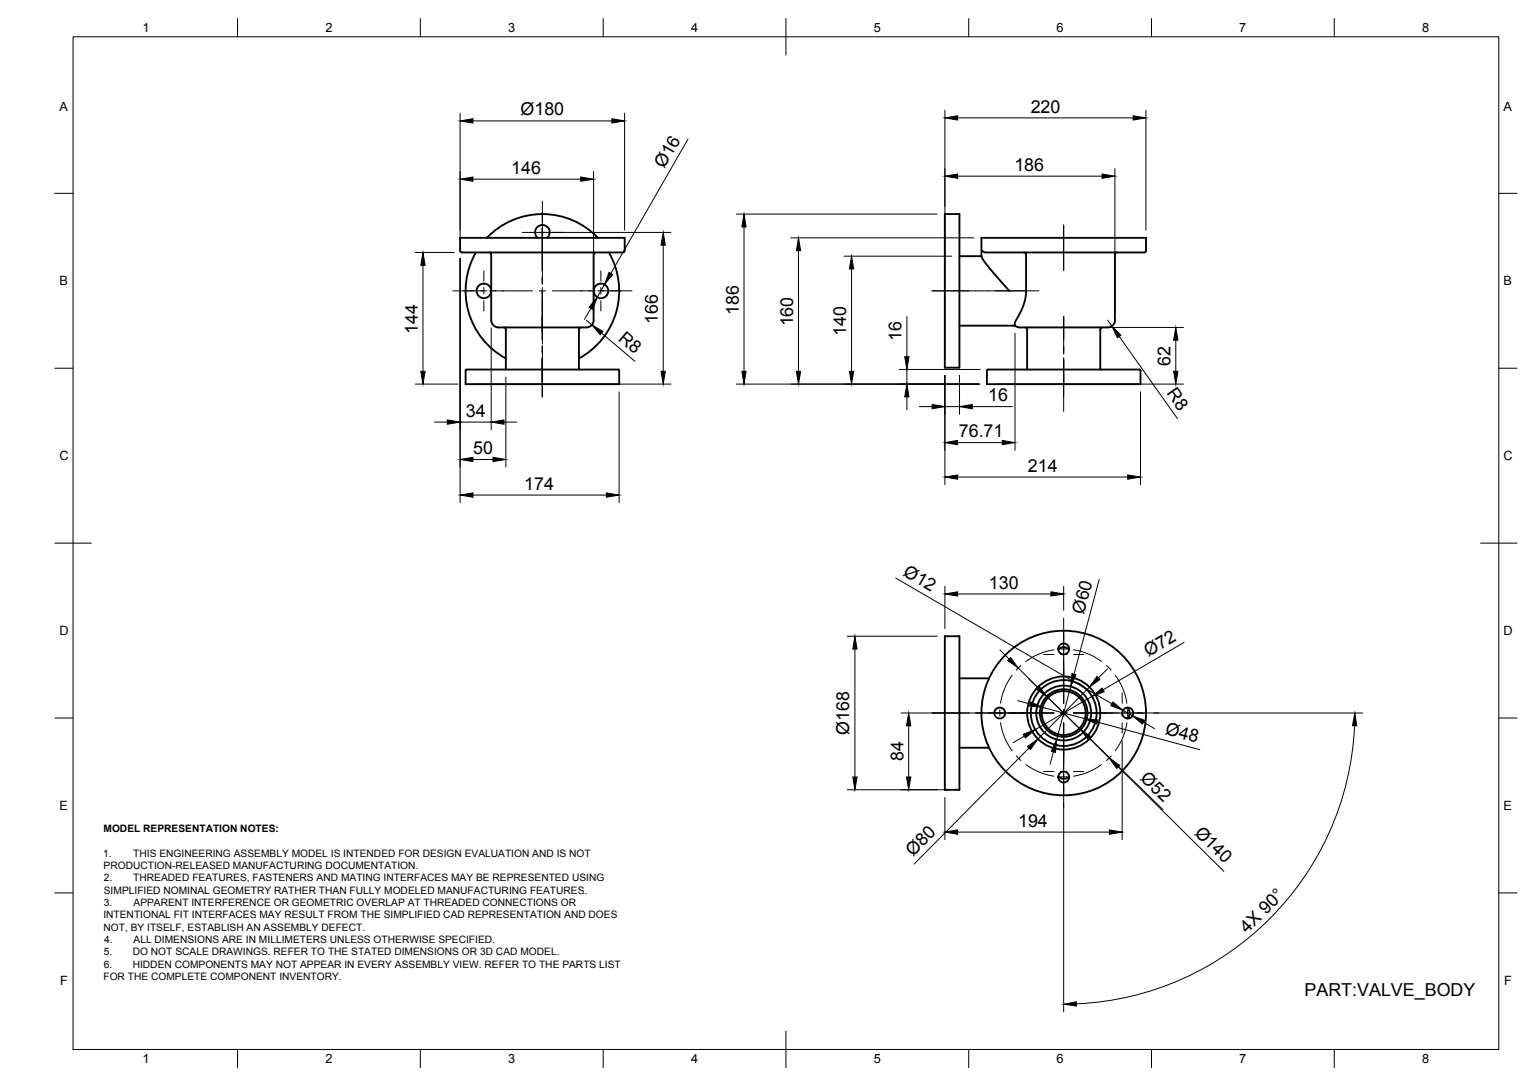
ISO-10303-21;
HEADER;
/* Generated by software containing ST-Developer
 * from STEP Tools, Inc. (www.steptools.com) 
 */

FILE_DESCRIPTION(
/* description */ (''),
/* implementation_level */ '2;1');

FILE_NAME(
/* name */ 'VALVE_BODY.step',
/* time_stamp */ '2026-10-04T02:10:06-07:00',
/* author */ (''),
/* organization */ (''),
/* preprocessor_version */ 'ST-DEVELOPER v20.2',
/* originating_system */ 'Autodesk Translation Framework v15.15.0.0',
/* authorisation */ '');

FILE_SCHEMA (('AUTOMOTIVE_DESIGN { 1 0 10303 214 3 1 1 }'));
ENDSEC;

DATA;
#10=MECHANICAL_DESIGN_GEOMETRIC_PRESENTATION_REPRESENTATION('',(#141),#9668);
#119=SHAPE_REPRESENTATION_RELATIONSHIP('SRR','None',#9712,#130);
#130=ADVANCED_BREP_SHAPE_REPRESENTATION('',(#152),#9657);
#141=STYLED_ITEM('',(#9775),#152);
#152=MANIFOLD_SOLID_BREP('Body1',#3881);
#163=CONICAL_SURFACE('',#4037,30.,0.785398163397447);
#164=CONICAL_SURFACE('',#4125,1000.,1.02974425867666);
#195=FACE_BOUND('',#1037,.T.);
#196=FACE_BOUND('',#1038,.T.);
#197=FACE_BOUND('',#1039,.T.);
#198=FACE_BOUND('',#1041,.T.);
#199=FACE_BOUND('',#1045,.T.);
#200=FACE_BOUND('',#1048,.T.);
#201=FACE_BOUND('',#1049,.T.);
#202=FACE_BOUND('',#1050,.T.);
#203=FACE_BOUND('',#1051,.T.);
#204=FACE_BOUND('',#1052,.T.);
#205=FACE_BOUND('',#1055,.T.);
#206=FACE_BOUND('',#1056,.T.);
#207=FACE_BOUND('',#1057,.T.);
#208=FACE_BOUND('',#1058,.T.);
#209=FACE_BOUND('',#1059,.T.);
#210=FACE_BOUND('',#1063,.T.);
#211=FACE_BOUND('',#1068,.T.);
#212=FACE_BOUND('',#1069,.T.);
#213=FACE_BOUND('',#1070,.T.);
#214=FACE_BOUND('',#1071,.T.);
#215=FACE_BOUND('',#1072,.T.);
#216=FACE_BOUND('',#1075,.T.);
#217=FACE_BOUND('',#1077,.T.);
#218=FACE_BOUND('',#1079,.T.);
#219=FACE_BOUND('',#1083,.T.);
#220=FACE_BOUND('',#1084,.T.);
#221=FACE_BOUND('',#1085,.T.);
#222=FACE_BOUND('',#1086,.T.);
#223=FACE_BOUND('',#1087,.T.);
#224=FACE_BOUND('',#1089,.T.);
#225=FACE_BOUND('',#1090,.T.);
#226=FACE_BOUND('',#1091,.T.);
#227=FACE_BOUND('',#1092,.T.);
#228=FACE_BOUND('',#1093,.T.);
#268=PLANE('',#4028);
#269=PLANE('',#4034);
#270=PLANE('',#4042);
#271=PLANE('',#4046);
#272=PLANE('',#4055);
#273=PLANE('',#4068);
#274=PLANE('',#4078);
#275=PLANE('',#4088);
#276=PLANE('',#4092);
#277=PLANE('',#4099);
#278=PLANE('',#4104);
#279=PLANE('',#4111);
#280=PLANE('',#4112);
#371=LINE('',#5637,#562);
#372=LINE('',#5688,#563);
#373=LINE('',#5690,#564);
#374=LINE('',#5995,#565);
#375=LINE('',#5997,#566);
#376=LINE('',#6015,#567);
#377=LINE('',#6018,#568);
#378=LINE('',#6025,#569);
#379=LINE('',#6040,#570);
#380=LINE('',#6059,#571);
#381=LINE('',#6078,#572);
#382=LINE('',#6080,#573);
#383=LINE('',#6082,#574);
#384=LINE('',#6084,#575);
#385=LINE('',#6102,#576);
#386=LINE('',#6109,#577);
#387=LINE('',#6190,#578);
#388=LINE('',#6213,#579);
#389=LINE('',#6214,#580);
#390=LINE('',#6216,#581);
#391=LINE('',#6218,#582);
#392=LINE('',#6220,#583);
#393=LINE('',#6222,#584);
#394=LINE('',#6224,#585);
#395=LINE('',#6226,#586);
#396=LINE('',#6228,#587);
#397=LINE('',#6230,#588);
#398=LINE('',#6232,#589);
#399=LINE('',#6234,#590);
#400=LINE('',#6236,#591);
#401=LINE('',#6239,#592);
#402=LINE('',#6245,#593);
#403=LINE('',#6247,#594);
#404=LINE('',#6249,#595);
#405=LINE('',#6251,#596);
#562=VECTOR('',#4483,18.3303029094034);
#563=VECTOR('',#4484,38.);
#564=VECTOR('',#4487,18.3303193041542);
#565=VECTOR('',#4504,15.6464703888607);
#566=VECTOR('',#4505,15.6464703888607);
#567=VECTOR('',#4526,30.);
#568=VECTOR('',#4529,26.);
#569=VECTOR('',#4538,23.9999999999998);
#570=VECTOR('',#4555,83.9999999999998);
#571=VECTOR('',#4576,39.9999999999999);
#572=VECTOR('',#4603,56.0000000000001);
#573=VECTOR('',#4606,7.94448724536034);
#574=VECTOR('',#4607,90.0000000000003);
#575=VECTOR('',#4610,7.94448724536034);
#576=VECTOR('',#4629,39.999999999998);
#577=VECTOR('',#4638,44.0000000000001);
#578=VECTOR('',#4653,84.);
#579=VECTOR('',#4680,40.0090835271346);
#580=VECTOR('',#4681,40.011431530049);
#581=VECTOR('',#4684,42.);
#582=VECTOR('',#4687,42.);
#583=VECTOR('',#4690,24.);
#584=VECTOR('',#4693,8.);
#585=VECTOR('',#4696,8.);
#586=VECTOR('',#4699,8.);
#587=VECTOR('',#4702,8.);
#588=VECTOR('',#4705,8.);
#589=VECTOR('',#4708,8.);
#590=VECTOR('',#4711,8.);
#591=VECTOR('',#4714,8.);
#592=VECTOR('',#4717,6.00000000000001);
#593=VECTOR('',#4724,1000.);
#594=VECTOR('',#4727,6.00000000000001);
#595=VECTOR('',#4730,6.00000000000001);
#596=VECTOR('',#4733,6.00000000000001);
#753=CYLINDRICAL_SURFACE('',#4020,38.);
#754=CYLINDRICAL_SURFACE('',#4040,26.);
#755=CYLINDRICAL_SURFACE('',#4044,23.9999999999998);
#756=CYLINDRICAL_SURFACE('',#4052,83.9999999999998);
#757=CYLINDRICAL_SURFACE('',#4062,39.9999999999999);
#758=CYLINDRICAL_SURFACE('',#4075,56.0000000000001);
#759=CYLINDRICAL_SURFACE('',#4076,90.0000000000003);
#760=CYLINDRICAL_SURFACE('',#4084,39.999999999998);
#761=CYLINDRICAL_SURFACE('',#4090,44.0000000000001);
#762=CYLINDRICAL_SURFACE('',#4096,84.);
#763=CYLINDRICAL_SURFACE('',#4110,56.);
#764=CYLINDRICAL_SURFACE('',#4113,24.);
#765=CYLINDRICAL_SURFACE('',#4114,8.);
#766=CYLINDRICAL_SURFACE('',#4115,8.);
#767=CYLINDRICAL_SURFACE('',#4116,8.);
#768=CYLINDRICAL_SURFACE('',#4117,8.);
#769=CYLINDRICAL_SURFACE('',#4118,8.);
#770=CYLINDRICAL_SURFACE('',#4119,8.);
#771=CYLINDRICAL_SURFACE('',#4120,8.);
#772=CYLINDRICAL_SURFACE('',#4121,8.);
#773=CYLINDRICAL_SURFACE('',#4122,6.00000000000001);
#774=CYLINDRICAL_SURFACE('',#4126,6.00000000000001);
#775=CYLINDRICAL_SURFACE('',#4127,6.00000000000001);
#776=CYLINDRICAL_SURFACE('',#4128,6.00000000000001);
#777=CYLINDRICAL_SURFACE('',#4129,30.);
#778=CYLINDRICAL_SURFACE('',#4130,30.);
#810=FACE_OUTER_BOUND('',#1033,.T.);
#811=FACE_OUTER_BOUND('',#1034,.T.);
#812=FACE_OUTER_BOUND('',#1035,.T.);
#813=FACE_OUTER_BOUND('',#1036,.T.);
#814=FACE_OUTER_BOUND('',#1040,.T.);
#815=FACE_OUTER_BOUND('',#1042,.T.);
#816=FACE_OUTER_BOUND('',#1043,.T.);
#817=FACE_OUTER_BOUND('',#1044,.T.);
#818=FACE_OUTER_BOUND('',#1046,.T.);
#819=FACE_OUTER_BOUND('',#1047,.T.);
#820=FACE_OUTER_BOUND('',#1053,.T.);
#821=FACE_OUTER_BOUND('',#1054,.T.);
#822=FACE_OUTER_BOUND('',#1060,.T.);
#823=FACE_OUTER_BOUND('',#1061,.T.);
#824=FACE_OUTER_BOUND('',#1062,.T.);
#825=FACE_OUTER_BOUND('',#1064,.T.);
#826=FACE_OUTER_BOUND('',#1065,.T.);
#827=FACE_OUTER_BOUND('',#1066,.T.);
#828=FACE_OUTER_BOUND('',#1067,.T.);
#829=FACE_OUTER_BOUND('',#1073,.T.);
#830=FACE_OUTER_BOUND('',#1074,.T.);
#831=FACE_OUTER_BOUND('',#1076,.T.);
#832=FACE_OUTER_BOUND('',#1078,.T.);
#833=FACE_OUTER_BOUND('',#1080,.T.);
#834=FACE_OUTER_BOUND('',#1081,.T.);
#835=FACE_OUTER_BOUND('',#1082,.T.);
#836=FACE_OUTER_BOUND('',#1088,.T.);
#837=FACE_OUTER_BOUND('',#1094,.T.);
#838=FACE_OUTER_BOUND('',#1095,.T.);
#839=FACE_OUTER_BOUND('',#1096,.T.);
#840=FACE_OUTER_BOUND('',#1097,.T.);
#841=FACE_OUTER_BOUND('',#1098,.T.);
#842=FACE_OUTER_BOUND('',#1099,.T.);
#843=FACE_OUTER_BOUND('',#1100,.T.);
#844=FACE_OUTER_BOUND('',#1101,.T.);
#845=FACE_OUTER_BOUND('',#1102,.T.);
#846=FACE_OUTER_BOUND('',#1103,.T.);
#847=FACE_OUTER_BOUND('',#1104,.T.);
#848=FACE_OUTER_BOUND('',#1105,.T.);
#849=FACE_OUTER_BOUND('',#1106,.T.);
#850=FACE_OUTER_BOUND('',#1107,.T.);
#851=FACE_OUTER_BOUND('',#1108,.T.);
#852=FACE_OUTER_BOUND('',#1109,.T.);
#853=FACE_OUTER_BOUND('',#1110,.T.);
#854=FACE_OUTER_BOUND('',#1111,.T.);
#855=FACE_OUTER_BOUND('',#1112,.T.);
#856=FACE_OUTER_BOUND('',#1113,.T.);
#857=FACE_OUTER_BOUND('',#1114,.T.);
#1033=EDGE_LOOP('',(#2541,#2542,#2543,#2544,#2545));
#1034=EDGE_LOOP('',(#2546,#2547,#2548,#2549,#2550,#2551,#2552,#2553,#2554,
#2555,#2556,#2557));
#1035=EDGE_LOOP('',(#2558,#2559,#2560,#2561,#2562,#2563,#2564,#2565,#2566));
#1036=EDGE_LOOP('',(#2567,#2568,#2569,#2570,#2571,#2572,#2573));
#1037=EDGE_LOOP('',(#2574));
#1038=EDGE_LOOP('',(#2575));
#1039=EDGE_LOOP('',(#2576));
#1040=EDGE_LOOP('',(#2577));
#1041=EDGE_LOOP('',(#2578));
#1042=EDGE_LOOP('',(#2579,#2580,#2581,#2582,#2583));
#1043=EDGE_LOOP('',(#2584,#2585,#2586,#2587,#2588));
#1044=EDGE_LOOP('',(#2589));
#1045=EDGE_LOOP('',(#2590));
#1046=EDGE_LOOP('',(#2591,#2592,#2593,#2594));
#1047=EDGE_LOOP('',(#2595));
#1048=EDGE_LOOP('',(#2596));
#1049=EDGE_LOOP('',(#2597));
#1050=EDGE_LOOP('',(#2598));
#1051=EDGE_LOOP('',(#2599));
#1052=EDGE_LOOP('',(#2600));
#1053=EDGE_LOOP('',(#2601,#2602,#2603,#2604,#2605));
#1054=EDGE_LOOP('',(#2606));
#1055=EDGE_LOOP('',(#2607));
#1056=EDGE_LOOP('',(#2608));
#1057=EDGE_LOOP('',(#2609));
#1058=EDGE_LOOP('',(#2610));
#1059=EDGE_LOOP('',(#2611));
#1060=EDGE_LOOP('',(#2612,#2613,#2614,#2615,#2616));
#1061=EDGE_LOOP('',(#2617,#2618,#2619,#2620,#2621));
#1062=EDGE_LOOP('',(#2622));
#1063=EDGE_LOOP('',(#2623));
#1064=EDGE_LOOP('',(#2624,#2625,#2626,#2627,#2628,#2629,#2630));
#1065=EDGE_LOOP('',(#2631,#2632,#2633,#2634,#2635,#2636,#2637,#2638,#2639));
#1066=EDGE_LOOP('',(#2640,#2641,#2642,#2643,#2644,#2645,#2646,#2647));
#1067=EDGE_LOOP('',(#2648));
#1068=EDGE_LOOP('',(#2649));
#1069=EDGE_LOOP('',(#2650));
#1070=EDGE_LOOP('',(#2651));
#1071=EDGE_LOOP('',(#2652));
#1072=EDGE_LOOP('',(#2653));
#1073=EDGE_LOOP('',(#2654,#2655,#2656,#2657,#2658));
#1074=EDGE_LOOP('',(#2659));
#1075=EDGE_LOOP('',(#2660));
#1076=EDGE_LOOP('',(#2661,#2662,#2663,#2664));
#1077=EDGE_LOOP('',(#2665,#2666));
#1078=EDGE_LOOP('',(#2667));
#1079=EDGE_LOOP('',(#2668));
#1080=EDGE_LOOP('',(#2669,#2670,#2671,#2672));
#1081=EDGE_LOOP('',(#2673,#2674,#2675,#2676));
#1082=EDGE_LOOP('',(#2677));
#1083=EDGE_LOOP('',(#2678));
#1084=EDGE_LOOP('',(#2679));
#1085=EDGE_LOOP('',(#2680));
#1086=EDGE_LOOP('',(#2681));
#1087=EDGE_LOOP('',(#2682));
#1088=EDGE_LOOP('',(#2683));
#1089=EDGE_LOOP('',(#2684));
#1090=EDGE_LOOP('',(#2685));
#1091=EDGE_LOOP('',(#2686));
#1092=EDGE_LOOP('',(#2687));
#1093=EDGE_LOOP('',(#2688));
#1094=EDGE_LOOP('',(#2689,#2690,#2691,#2692));
#1095=EDGE_LOOP('',(#2693,#2694,#2695,#2696,#2697));
#1096=EDGE_LOOP('',(#2698,#2699,#2700,#2701,#2702));
#1097=EDGE_LOOP('',(#2703,#2704,#2705,#2706,#2707));
#1098=EDGE_LOOP('',(#2708,#2709,#2710,#2711));
#1099=EDGE_LOOP('',(#2712,#2713,#2714,#2715));
#1100=EDGE_LOOP('',(#2716,#2717,#2718,#2719));
#1101=EDGE_LOOP('',(#2720,#2721,#2722,#2723));
#1102=EDGE_LOOP('',(#2724,#2725,#2726,#2727));
#1103=EDGE_LOOP('',(#2728,#2729,#2730,#2731));
#1104=EDGE_LOOP('',(#2732,#2733,#2734,#2735));
#1105=EDGE_LOOP('',(#2736,#2737,#2738,#2739));
#1106=EDGE_LOOP('',(#2740,#2741,#2742,#2743,#2744));
#1107=EDGE_LOOP('',(#2745,#2746,#2747,#2748));
#1108=EDGE_LOOP('',(#2749,#2750,#2751,#2752));
#1109=EDGE_LOOP('',(#2753,#2754,#2755,#2756));
#1110=EDGE_LOOP('',(#2757,#2758,#2759,#2760));
#1111=EDGE_LOOP('',(#2761,#2762,#2763,#2764,#2765));
#1112=EDGE_LOOP('',(#2766,#2767,#2768,#2769,#2770));
#1113=EDGE_LOOP('',(#2771,#2772,#2773,#2774,#2775));
#1114=EDGE_LOOP('',(#2776,#2777,#2778,#2779,#2780));
#1329=B_SPLINE_CURVE_WITH_KNOTS('',3,(#5577,#5578,#5579,#5580,#5581,#5582,
#5583,#5584),.UNSPECIFIED.,.F.,.F.,(4,2,2,4),(-1.5505171028707,-1.25408209125058,
0.,0.00304904819120853),.UNSPECIFIED.);
#1330=B_SPLINE_CURVE_WITH_KNOTS('',3,(#5589,#5590,#5591,#5592,#5593,#5594,
#5595,#5596,#5597,#5598),.UNSPECIFIED.,.F.,.F.,(4,2,2,2,4),(4.80501349520982,
5.06951274232393,5.98994668417101,6.94716893318789,6.95166465756746),
 .UNSPECIFIED.);
#1331=B_SPLINE_CURVE_WITH_KNOTS('',3,(#5602,#5603,#5604,#5605,#5606,#5607,
#5608,#5609,#5610,#5611,#5612,#5613,#5614,#5615,#5616,#5617,#5618,#5619,
#5620,#5621,#5622,#5623,#5624,#5625,#5626,#5627,#5628,#5629,#5630,#5631,
#5632,#5633,#5634,#5635),.UNSPECIFIED.,.F.,.F.,(4,2,2,2,2,2,2,2,2,2,2,2,
2,2,2,2,4),(11.9511654991448,12.7026512908879,13.4541370826309,14.205622874374,
14.9571086661171,15.6995186161844,16.4419285662517,17.184338516319,17.9267484663863,
18.6691583423927,19.4115682183991,20.1539780944055,20.8963879704119,21.6478737273813,
22.3993594843507,23.1508452413201,23.9023309982895),.UNSPECIFIED.);
#1332=B_SPLINE_CURVE_WITH_KNOTS('',3,(#5639,#5640,#5641,#5642,#5643,#5644,
#5645,#5646,#5647,#5648,#5649,#5650,#5651,#5652,#5653,#5654,#5655,#5656),
 .UNSPECIFIED.,.F.,.F.,(4,2,2,2,2,2,2,2,4),(15.4947128296219,15.6730696180795,
16.2614804512611,16.8498912844427,17.4383021176243,18.3068888332102,19.1754755487961,
20.0440622643819,20.9126489799678),.UNSPECIFIED.);
#1333=B_SPLINE_CURVE_WITH_KNOTS('',3,(#5658,#5659,#5660,#5661,#5662,#5663,
#5664,#5665,#5666,#5667),.UNSPECIFIED.,.F.,.F.,(4,2,2,2,4),(-6.98864961225109,
-6.53092622927509,-5.80568103754781,-5.08043584582052,-4.62271246284453),
 .UNSPECIFIED.);
#1334=B_SPLINE_CURVE_WITH_KNOTS('',3,(#5669,#5670,#5671,#5672,#5673,#5674,
#5675,#5676,#5677,#5678,#5679,#5680,#5681,#5682,#5683,#5684,#5685,#5686),
 .UNSPECIFIED.,.F.,.F.,(4,2,2,2,2,2,2,2,4),(-5.41793615034587,-5.23957936188825,
-4.65116852870664,-4.06275769552503,-3.47434686234343,-2.60576014675757,
-1.73717343117172,-0.868586715585868,-1.50990331349021E-14),
 .UNSPECIFIED.);
#1335=B_SPLINE_CURVE_WITH_KNOTS('',3,(#5692,#5693,#5694,#5695,#5696,#5697,
#5698,#5699,#5700,#5701,#5702,#5703,#5704,#5705),.UNSPECIFIED.,.F.,.F.,
(4,2,2,2,2,2,4),(0.,0.75148577435623,1.50297154871246,2.25445732306868,
3.00594309742491,3.74835301046176,3.85208753126486),.UNSPECIFIED.);
#1336=B_SPLINE_CURVE_WITH_KNOTS('',3,(#5707,#5708,#5709,#5710,#5711,#5712,
#5713,#5714,#5715,#5716,#5717,#5718,#5719,#5720,#5721,#5722,#5723,#5724,
#5725,#5726,#5727,#5728),.UNSPECIFIED.,.F.,.F.,(4,2,2,2,2,2,2,2,2,2,4),
(1.02020510036039E-13,0.836743409431383,1.52319262533783,1.73458721528613,
1.86686045602122,1.99232796114447,2.16705857121117,2.37875039685339,2.77213838176281,
3.6146168888541,3.63735578863517),.UNSPECIFIED.);
#1337=B_SPLINE_CURVE_WITH_KNOTS('',3,(#5729,#5730,#5731,#5732,#5733,#5734,
#5735,#5736,#5737,#5738,#5739,#5740,#5741,#5742,#5743,#5744,#5745,#5746,
#5747,#5748,#5749,#5750,#5751,#5752,#5753,#5754,#5755,#5756,#5757,#5758,
#5759,#5760,#5761,#5762,#5763,#5764,#5765,#5766,#5767,#5768,#5769,#5770,
#5771,#5772,#5773,#5774),.UNSPECIFIED.,.F.,.F.,(4,2,2,2,2,2,2,2,2,2,2,2,
2,2,2,2,2,2,2,2,2,2,4),(-15.8032530304094,-15.6995185096063,-14.9571085965695,
-14.2056228222133,-13.454137047857,-12.7026512735008,-11.9511654991446,
-11.1996797247884,-10.4481939504321,-9.6967081760759,-8.94522240171967,
-8.20281248868283,-7.46040257564598,-6.71799266260913,-5.97558274957229,
-5.23317283653545,-4.4907629234986,-3.74835301046175,-3.00594309742491,
-2.25445732306868,-1.50297154871245,-0.751485774356227,0.),
 .UNSPECIFIED.);
#1338=B_SPLINE_CURVE_WITH_KNOTS('',3,(#5785,#5786,#5787,#5788,#5789,#5790,
#5791,#5792,#5793,#5794),.UNSPECIFIED.,.F.,.F.,(4,2,2,2,4),(-1.04015949094204,
-0.932657377635769,-0.838016147397311,-0.758953484458178,-0.692999614147385),
 .UNSPECIFIED.);
#1339=B_SPLINE_CURVE_WITH_KNOTS('',3,(#5796,#5797,#5798,#5799,#5800,#5801,
#5802,#5803,#5804,#5805,#5806,#5807,#5808,#5809,#5810,#5811,#5812,#5813,
#5814,#5815,#5816,#5817,#5818,#5819,#5820,#5821,#5822,#5823,#5824,#5825,
#5826,#5827,#5828,#5829,#5830,#5831,#5832,#5833,#5834,#5835,#5836,#5837,
#5838,#5839,#5840,#5841,#5842,#5843,#5844,#5845,#5846,#5847,#5848,#5849,
#5850,#5851,#5852,#5853,#5854,#5855,#5856,#5857,#5858,#5859,#5860,#5861,
#5862,#5863,#5864,#5865,#5866,#5867,#5868,#5869,#5870,#5871,#5872,#5873,
#5874,#5875,#5876,#5877,#5878,#5879,#5880,#5881,#5882,#5883,#5884,#5885,
#5886,#5887,#5888,#5889,#5890,#5891,#5892,#5893,#5894,#5895,#5896,#5897,
#5898,#5899,#5900,#5901,#5902,#5903,#5904,#5905,#5906,#5907,#5908,#5909,
#5910,#5911,#5912,#5913,#5914,#5915,#5916,#5917,#5918,#5919,#5920,#5921,
#5922,#5923,#5924,#5925,#5926,#5927,#5928,#5929,#5930,#5931,#5932,#5933,
#5934,#5935,#5936,#5937,#5938,#5939,#5940,#5941,#5942,#5943,#5944,#5945,
#5946,#5947,#5948,#5949,#5950,#5951,#5952,#5953,#5954,#5955,#5956,#5957,
#5958,#5959,#5960,#5961,#5962,#5963,#5964,#5965,#5966,#5967,#5968,#5969,
#5970,#5971,#5972,#5973,#5974,#5975,#5976,#5977,#5978,#5979),
 .UNSPECIFIED.,.F.,.F.,(4,3,3,3,3,3,3,3,3,3,3,3,3,3,3,3,3,3,3,3,3,3,3,3,
3,3,3,3,3,3,3,3,3,3,3,3,3,3,3,3,3,3,3,3,3,3,3,3,3,3,3,3,3,3,3,3,3,3,3,3,
3,4),(2.72107972055907E-7,0.00178477543725798,0.00262815346851988,0.00401562885331435,
0.00525603482906771,0.00723037697612098,0.00921337722618793,0.0105117975501634,
0.0126012160788207,0.0131396789107112,0.0155870223193016,0.015767560271259,
0.0173527198466303,0.0183954416318069,0.0196367719226344,0.0208775813990201,
0.0210233229923547,0.0236512043529025,0.0255955755957421,0.0262790857134503,
0.0283626428282405,0.0304454519035474,0.031534848434546,0.0338165992760133,
0.0341627297950938,0.0354766704753677,0.036506599524544,0.0367906111556417,
0.0386488000158229,0.0394184925161895,0.0412258034154853,0.0420463738767373,
0.0442437218200704,0.0446742552372851,0.0467464838413529,0.047302136597833,
0.0493898024917242,0.0499300179583808,0.0520165802882478,0.0525578993189286,
0.0544927525372392,0.0551857806794765,0.0561500246532634,0.0564997213597504,
0.0578136620400243,0.060038018841681,0.0604415434005721,0.0624671007693764,
0.0630694247611199,0.0652001506910268,0.0673302255123812,0.0683251874822156,
0.0702926229698116,0.0722499651986351,0.0735809502033112,0.0748948908835851,
0.0762088315638591,0.0779650853238908,0.0788367129244069,0.0809688957796963,
0.0830959029701868,0.0840924756455026),.UNSPECIFIED.);
#1340=B_SPLINE_CURVE_WITH_KNOTS('',3,(#5981,#5982,#5983,#5984,#5985,#5986,
#5987,#5988,#5989,#5990),.UNSPECIFIED.,.F.,.F.,(4,2,2,2,4),(-0.69090250484878,
-0.624714986528312,-0.545652323589179,-0.45101109335072,-0.34350898004445),
 .UNSPECIFIED.);
#1341=B_SPLINE_CURVE_WITH_KNOTS('',3,(#6113,#6114,#6115,#6116,#6117,#6118,
#6119,#6120,#6121,#6122,#6123,#6124,#6125,#6126,#6127,#6128,#6129,#6130,
#6131,#6132,#6133,#6134,#6135,#6136,#6137,#6138,#6139,#6140,#6141,#6142,
#6143,#6144,#6145,#6146),.UNSPECIFIED.,.F.,.F.,(4,2,2,2,2,2,2,2,2,2,2,2,
2,2,2,2,4),(7.41376519068543,7.87807291581701,8.34238064094858,8.80668836608016,
9.27099609121173,9.73340901491583,10.1958219386199,10.658234862324,11.1206477860281,
11.5830607097322,12.0454736334363,12.5078865571404,12.9702994808445,13.4346072059761,
13.8989149311077,14.3632226562393,14.8275303813708),.UNSPECIFIED.);
#1342=B_SPLINE_CURVE_WITH_KNOTS('',3,(#6147,#6148,#6149,#6150,#6151,#6152,
#6153,#6154,#6155,#6156,#6157,#6158,#6159,#6160,#6161,#6162,#6163,#6164,
#6165,#6166,#6167,#6168,#6169,#6170,#6171,#6172,#6173,#6174,#6175,#6176,
#6177,#6178,#6179,#6180),.UNSPECIFIED.,.F.,.F.,(4,2,2,2,2,2,2,2,2,2,2,2,
2,2,2,2,4),(14.8275303813708,15.2918381065024,15.756145831634,16.2204535567656,
16.6847612818971,17.1471742056012,17.6095871293054,18.0720000530095,18.5344129767136,
18.9968259004177,19.4592388241218,19.9216517478259,20.38406467153,20.8483723966616,
21.3126801217931,21.7769878469247,22.2412955720563),.UNSPECIFIED.);
#1427=CIRCLE('',#4017,88.0000000000002);
#1428=CIRCLE('',#4018,90.0000000000002);
#1429=CIRCLE('',#4019,90.0000000000002);
#1430=CIRCLE('',#4021,38.);
#1431=CIRCLE('',#4023,56.0000000000002);
#1432=CIRCLE('',#4024,56.0000000000002);
#1433=CIRCLE('',#4025,2.);
#1434=CIRCLE('',#4026,58.0000000000002);
#1435=CIRCLE('',#4027,58.0000000000002);
#1436=CIRCLE('',#4029,30.);
#1437=CIRCLE('',#4030,30.);
#1438=CIRCLE('',#4031,6.00000000000001);
#1439=CIRCLE('',#4032,6.00000000000001);
#1440=CIRCLE('',#4033,6.00000000000001);
#1441=CIRCLE('',#4035,36.);
#1442=CIRCLE('',#4036,30.);
#1443=CIRCLE('',#4038,26.);
#1444=CIRCLE('',#4039,26.);
#1445=CIRCLE('',#4041,25.9999999999999);
#1446=CIRCLE('',#4043,23.9999999999999);
#1447=CIRCLE('',#4045,23.9999999999997);
#1448=CIRCLE('',#4047,83.9999999999997);
#1449=CIRCLE('',#4048,8.);
#1450=CIRCLE('',#4049,8.);
#1451=CIRCLE('',#4050,8.);
#1452=CIRCLE('',#4051,8.);
#1453=CIRCLE('',#4053,83.9999999999998);
#1454=CIRCLE('',#4054,83.9999999999998);
#1455=CIRCLE('',#4056,82.9999999999998);
#1456=CIRCLE('',#4057,8.);
#1457=CIRCLE('',#4058,8.);
#1458=CIRCLE('',#4059,8.);
#1459=CIRCLE('',#4060,8.);
#1460=CIRCLE('',#4061,39.9999999999998);
#1461=CIRCLE('',#4063,39.9999999999999);
#1462=CIRCLE('',#4064,39.9999999999999);
#1463=CIRCLE('',#4066,2.);
#1464=CIRCLE('',#4067,42.);
#1465=CIRCLE('',#4069,47.9999999999999);
#1466=CIRCLE('',#4071,8.);
#1467=CIRCLE('',#4072,56.);
#1468=CIRCLE('',#4073,56.);
#1469=CIRCLE('',#4074,56.);
#1470=CIRCLE('',#4077,90.0000000000003);
#1471=CIRCLE('',#4079,40.999999999998);
#1472=CIRCLE('',#4080,6.00000000000001);
#1473=CIRCLE('',#4081,6.00000000000001);
#1474=CIRCLE('',#4082,6.00000000000001);
#1475=CIRCLE('',#4083,6.00000000000001);
#1476=CIRCLE('',#4085,39.999999999998);
#1477=CIRCLE('',#4086,39.999999999998);
#1478=CIRCLE('',#4087,39.999999999998);
#1479=CIRCLE('',#4089,44.0000000000002);
#1480=CIRCLE('',#4091,44.);
#1481=CIRCLE('',#4093,38.5);
#1482=CIRCLE('',#4095,2.5);
#1483=CIRCLE('',#4097,84.);
#1484=CIRCLE('',#4098,84.);
#1485=CIRCLE('',#4100,8.);
#1486=CIRCLE('',#4101,8.);
#1487=CIRCLE('',#4102,8.);
#1488=CIRCLE('',#4103,8.);
#1489=CIRCLE('',#4105,8.);
#1490=CIRCLE('',#4106,8.);
#1491=CIRCLE('',#4107,8.);
#1492=CIRCLE('',#4108,8.);
#1493=CIRCLE('',#4109,24.);
#1494=CIRCLE('',#4123,6.00000000000002);
#1495=CIRCLE('',#4124,6.00000000000002);
#1496=CIRCLE('',#4132,1.);
#1497=CIRCLE('',#4134,1.);
#1641=VERTEX_POINT('',#5573);
#1642=VERTEX_POINT('',#5574);
#1643=VERTEX_POINT('',#5576);
#1644=VERTEX_POINT('',#5585);
#1645=VERTEX_POINT('',#5587);
#1646=VERTEX_POINT('',#5600);
#1647=VERTEX_POINT('',#5601);
#1648=VERTEX_POINT('',#5636);
#1649=VERTEX_POINT('',#5638);
#1650=VERTEX_POINT('',#5657);
#1651=VERTEX_POINT('',#5668);
#1652=VERTEX_POINT('',#5687);
#1653=VERTEX_POINT('',#5691);
#1654=VERTEX_POINT('',#5706);
#1655=VERTEX_POINT('',#5776);
#1656=VERTEX_POINT('',#5777);
#1657=VERTEX_POINT('',#5780);
#1658=VERTEX_POINT('',#5782);
#1659=VERTEX_POINT('',#5784);
#1660=VERTEX_POINT('',#5795);
#1661=VERTEX_POINT('',#5980);
#1662=VERTEX_POINT('',#5993);
#1663=VERTEX_POINT('',#5996);
#1664=VERTEX_POINT('',#5999);
#1665=VERTEX_POINT('',#6001);
#1666=VERTEX_POINT('',#6003);
#1667=VERTEX_POINT('',#6006);
#1668=VERTEX_POINT('',#6008);
#1669=VERTEX_POINT('',#6011);
#1670=VERTEX_POINT('',#6012);
#1671=VERTEX_POINT('',#6017);
#1672=VERTEX_POINT('',#6021);
#1673=VERTEX_POINT('',#6024);
#1674=VERTEX_POINT('',#6028);
#1675=VERTEX_POINT('',#6030);
#1676=VERTEX_POINT('',#6032);
#1677=VERTEX_POINT('',#6034);
#1678=VERTEX_POINT('',#6036);
#1679=VERTEX_POINT('',#6039);
#1680=VERTEX_POINT('',#6041);
#1681=VERTEX_POINT('',#6045);
#1682=VERTEX_POINT('',#6047);
#1683=VERTEX_POINT('',#6049);
#1684=VERTEX_POINT('',#6051);
#1685=VERTEX_POINT('',#6053);
#1686=VERTEX_POINT('',#6055);
#1687=VERTEX_POINT('',#6058);
#1688=VERTEX_POINT('',#6060);
#1689=VERTEX_POINT('',#6064);
#1690=VERTEX_POINT('',#6068);
#1691=VERTEX_POINT('',#6071);
#1692=VERTEX_POINT('',#6073);
#1693=VERTEX_POINT('',#6081);
#1694=VERTEX_POINT('',#6086);
#1695=VERTEX_POINT('',#6088);
#1696=VERTEX_POINT('',#6090);
#1697=VERTEX_POINT('',#6092);
#1698=VERTEX_POINT('',#6094);
#1699=VERTEX_POINT('',#6097);
#1700=VERTEX_POINT('',#6098);
#1701=VERTEX_POINT('',#6101);
#1702=VERTEX_POINT('',#6105);
#1703=VERTEX_POINT('',#6108);
#1704=VERTEX_POINT('',#6111);
#1705=VERTEX_POINT('',#6112);
#1706=VERTEX_POINT('',#6182);
#1707=VERTEX_POINT('',#6187);
#1708=VERTEX_POINT('',#6189);
#1709=VERTEX_POINT('',#6193);
#1710=VERTEX_POINT('',#6195);
#1711=VERTEX_POINT('',#6197);
#1712=VERTEX_POINT('',#6199);
#1713=VERTEX_POINT('',#6202);
#1714=VERTEX_POINT('',#6204);
#1715=VERTEX_POINT('',#6206);
#1716=VERTEX_POINT('',#6208);
#1717=VERTEX_POINT('',#6210);
#1718=VERTEX_POINT('',#6238);
#1719=VERTEX_POINT('',#6240);
#1720=VERTEX_POINT('',#6244);
#1994=EDGE_CURVE('',#1641,#1642,#1427,.T.);
#1995=EDGE_CURVE('',#1641,#1643,#1329,.T.);
#1996=EDGE_CURVE('',#1643,#1644,#1428,.T.);
#1997=EDGE_CURVE('',#1644,#1645,#1429,.T.);
#1998=EDGE_CURVE('',#1645,#1642,#1330,.F.);
#1999=EDGE_CURVE('',#1646,#1647,#1331,.T.);
#2000=EDGE_CURVE('',#1647,#1648,#371,.T.);
#2001=EDGE_CURVE('',#1648,#1649,#1332,.F.);
#2002=EDGE_CURVE('',#1649,#1650,#1333,.T.);
#2003=EDGE_CURVE('',#1650,#1651,#1334,.T.);
#2004=EDGE_CURVE('',#1652,#1651,#372,.T.);
#2005=EDGE_CURVE('',#1652,#1652,#1430,.F.);
#2006=EDGE_CURVE('',#1651,#1646,#373,.T.);
#2007=EDGE_CURVE('',#1646,#1653,#1335,.T.);
#2008=EDGE_CURVE('',#1653,#1654,#1336,.T.);
#2009=EDGE_CURVE('',#1654,#1646,#1337,.T.);
#2010=EDGE_CURVE('',#1655,#1656,#1431,.T.);
#2011=EDGE_CURVE('',#1656,#1655,#1432,.T.);
#2012=EDGE_CURVE('',#1656,#1657,#1433,.T.);
#2013=EDGE_CURVE('',#1657,#1658,#1434,.T.);
#2014=EDGE_CURVE('',#1658,#1659,#1338,.T.);
#2015=EDGE_CURVE('',#1659,#1660,#1339,.T.);
#2016=EDGE_CURVE('',#1660,#1661,#1340,.T.);
#2017=EDGE_CURVE('',#1661,#1657,#1435,.T.);
#2018=EDGE_CURVE('',#1642,#1662,#1436,.F.);
#2019=EDGE_CURVE('',#1658,#1662,#374,.T.);
#2020=EDGE_CURVE('',#1663,#1661,#375,.T.);
#2021=EDGE_CURVE('',#1663,#1641,#1437,.F.);
#2022=EDGE_CURVE('',#1664,#1664,#1438,.T.);
#2023=EDGE_CURVE('',#1665,#1665,#1439,.T.);
#2024=EDGE_CURVE('',#1666,#1666,#1440,.T.);
#2025=EDGE_CURVE('',#1667,#1667,#1441,.T.);
#2026=EDGE_CURVE('',#1668,#1668,#1442,.T.);
#2027=EDGE_CURVE('',#1669,#1670,#1443,.T.);
#2028=EDGE_CURVE('',#1670,#1669,#1444,.T.);
#2029=EDGE_CURVE('',#1669,#1668,#376,.T.);
#2030=EDGE_CURVE('',#1670,#1671,#377,.T.);
#2031=EDGE_CURVE('',#1671,#1671,#1445,.T.);
#2032=EDGE_CURVE('',#1672,#1672,#1446,.T.);
#2033=EDGE_CURVE('',#1672,#1673,#378,.T.);
#2034=EDGE_CURVE('',#1673,#1673,#1447,.T.);
#2035=EDGE_CURVE('',#1674,#1674,#1448,.T.);
#2036=EDGE_CURVE('',#1675,#1675,#1449,.T.);
#2037=EDGE_CURVE('',#1676,#1676,#1450,.T.);
#2038=EDGE_CURVE('',#1677,#1677,#1451,.T.);
#2039=EDGE_CURVE('',#1678,#1678,#1452,.T.);
#2040=EDGE_CURVE('',#1674,#1679,#379,.T.);
#2041=EDGE_CURVE('',#1679,#1680,#1453,.F.);
#2042=EDGE_CURVE('',#1680,#1679,#1454,.F.);
#2043=EDGE_CURVE('',#1681,#1681,#1455,.T.);
#2044=EDGE_CURVE('',#1682,#1682,#1456,.F.);
#2045=EDGE_CURVE('',#1683,#1683,#1457,.F.);
#2046=EDGE_CURVE('',#1684,#1684,#1458,.F.);
#2047=EDGE_CURVE('',#1685,#1685,#1459,.F.);
#2048=EDGE_CURVE('',#1686,#1686,#1460,.T.);
#2049=EDGE_CURVE('',#1686,#1687,#380,.T.);
#2050=EDGE_CURVE('',#1687,#1688,#1461,.T.);
#2051=EDGE_CURVE('',#1688,#1687,#1462,.T.);
#2052=EDGE_CURVE('',#1688,#1689,#1463,.T.);
#2053=EDGE_CURVE('',#1689,#1689,#1464,.T.);
#2054=EDGE_CURVE('',#1690,#1690,#1465,.T.);
#2055=EDGE_CURVE('',#1690,#1691,#1466,.T.);
#2056=EDGE_CURVE('',#1691,#1692,#1467,.T.);
#2057=EDGE_CURVE('',#1692,#1654,#1468,.T.);
#2058=EDGE_CURVE('',#1653,#1691,#1469,.T.);
#2059=EDGE_CURVE('',#1692,#1655,#381,.T.);
#2060=EDGE_CURVE('',#1649,#1645,#382,.F.);
#2061=EDGE_CURVE('',#1644,#1693,#383,.T.);
#2062=EDGE_CURVE('',#1693,#1693,#1470,.T.);
#2063=EDGE_CURVE('',#1643,#1650,#384,.T.);
#2064=EDGE_CURVE('',#1694,#1694,#1471,.F.);
#2065=EDGE_CURVE('',#1695,#1695,#1472,.T.);
#2066=EDGE_CURVE('',#1696,#1696,#1473,.T.);
#2067=EDGE_CURVE('',#1697,#1697,#1474,.T.);
#2068=EDGE_CURVE('',#1698,#1698,#1475,.T.);
#2069=EDGE_CURVE('',#1699,#1700,#1476,.T.);
#2070=EDGE_CURVE('',#1700,#1699,#1477,.T.);
#2071=EDGE_CURVE('',#1699,#1701,#385,.T.);
#2072=EDGE_CURVE('',#1701,#1701,#1478,.T.);
#2073=EDGE_CURVE('',#1702,#1702,#1479,.T.);
#2074=EDGE_CURVE('',#1702,#1703,#386,.T.);
#2075=EDGE_CURVE('',#1703,#1703,#1480,.T.);
#2076=EDGE_CURVE('',#1704,#1705,#1341,.T.);
#2077=EDGE_CURVE('',#1705,#1704,#1342,.T.);
#2078=EDGE_CURVE('',#1706,#1706,#1481,.T.);
#2079=EDGE_CURVE('',#1706,#1667,#1482,.T.);
#2080=EDGE_CURVE('',#1707,#1707,#1483,.T.);
#2081=EDGE_CURVE('',#1707,#1708,#387,.T.);
#2082=EDGE_CURVE('',#1708,#1708,#1484,.T.);
#2083=EDGE_CURVE('',#1709,#1709,#1485,.F.);
#2084=EDGE_CURVE('',#1710,#1710,#1486,.F.);
#2085=EDGE_CURVE('',#1711,#1711,#1487,.F.);
#2086=EDGE_CURVE('',#1712,#1712,#1488,.F.);
#2087=EDGE_CURVE('',#1713,#1713,#1489,.T.);
#2088=EDGE_CURVE('',#1714,#1714,#1490,.T.);
#2089=EDGE_CURVE('',#1715,#1715,#1491,.T.);
#2090=EDGE_CURVE('',#1716,#1716,#1492,.T.);
#2091=EDGE_CURVE('',#1717,#1717,#1493,.T.);
#2092=EDGE_CURVE('',#1646,#1660,#388,.T.);
#2093=EDGE_CURVE('',#1647,#1659,#389,.T.);
#2094=EDGE_CURVE('',#1662,#1648,#390,.F.);
#2095=EDGE_CURVE('',#1651,#1663,#391,.T.);
#2096=EDGE_CURVE('',#1705,#1717,#392,.T.);
#2097=EDGE_CURVE('',#1712,#1716,#393,.T.);
#2098=EDGE_CURVE('',#1711,#1715,#394,.T.);
#2099=EDGE_CURVE('',#1710,#1714,#395,.T.);
#2100=EDGE_CURVE('',#1709,#1713,#396,.T.);
#2101=EDGE_CURVE('',#1685,#1678,#397,.T.);
#2102=EDGE_CURVE('',#1684,#1677,#398,.T.);
#2103=EDGE_CURVE('',#1683,#1676,#399,.T.);
#2104=EDGE_CURVE('',#1682,#1675,#400,.T.);
#2105=EDGE_CURVE('',#1698,#1718,#401,.T.);
#2106=EDGE_CURVE('',#1718,#1719,#1494,.T.);
#2107=EDGE_CURVE('',#1719,#1718,#1495,.T.);
#2108=EDGE_CURVE('',#1720,#1719,#402,.T.);
#2109=EDGE_CURVE('',#1697,#1666,#403,.T.);
#2110=EDGE_CURVE('',#1696,#1665,#404,.T.);
#2111=EDGE_CURVE('',#1695,#1664,#405,.T.);
#2112=EDGE_CURVE('',#1700,#1694,#1496,.T.);
#2113=EDGE_CURVE('',#1681,#1680,#1497,.T.);
#2541=ORIENTED_EDGE('',*,*,#1994,.F.);
#2542=ORIENTED_EDGE('',*,*,#1995,.T.);
#2543=ORIENTED_EDGE('',*,*,#1996,.T.);
#2544=ORIENTED_EDGE('',*,*,#1997,.T.);
#2545=ORIENTED_EDGE('',*,*,#1998,.T.);
#2546=ORIENTED_EDGE('',*,*,#1999,.T.);
#2547=ORIENTED_EDGE('',*,*,#2000,.T.);
#2548=ORIENTED_EDGE('',*,*,#2001,.T.);
#2549=ORIENTED_EDGE('',*,*,#2002,.T.);
#2550=ORIENTED_EDGE('',*,*,#2003,.T.);
#2551=ORIENTED_EDGE('',*,*,#2004,.F.);
#2552=ORIENTED_EDGE('',*,*,#2005,.T.);
#2553=ORIENTED_EDGE('',*,*,#2004,.T.);
#2554=ORIENTED_EDGE('',*,*,#2006,.T.);
#2555=ORIENTED_EDGE('',*,*,#2007,.T.);
#2556=ORIENTED_EDGE('',*,*,#2008,.T.);
#2557=ORIENTED_EDGE('',*,*,#2009,.T.);
#2558=ORIENTED_EDGE('',*,*,#2010,.F.);
#2559=ORIENTED_EDGE('',*,*,#2011,.F.);
#2560=ORIENTED_EDGE('',*,*,#2012,.T.);
#2561=ORIENTED_EDGE('',*,*,#2013,.T.);
#2562=ORIENTED_EDGE('',*,*,#2014,.T.);
#2563=ORIENTED_EDGE('',*,*,#2015,.T.);
#2564=ORIENTED_EDGE('',*,*,#2016,.T.);
#2565=ORIENTED_EDGE('',*,*,#2017,.T.);
#2566=ORIENTED_EDGE('',*,*,#2012,.F.);
#2567=ORIENTED_EDGE('',*,*,#1994,.T.);
#2568=ORIENTED_EDGE('',*,*,#2018,.T.);
#2569=ORIENTED_EDGE('',*,*,#2019,.F.);
#2570=ORIENTED_EDGE('',*,*,#2013,.F.);
#2571=ORIENTED_EDGE('',*,*,#2017,.F.);
#2572=ORIENTED_EDGE('',*,*,#2020,.F.);
#2573=ORIENTED_EDGE('',*,*,#2021,.T.);
#2574=ORIENTED_EDGE('',*,*,#2022,.F.);
#2575=ORIENTED_EDGE('',*,*,#2023,.F.);
#2576=ORIENTED_EDGE('',*,*,#2024,.F.);
#2577=ORIENTED_EDGE('',*,*,#2025,.F.);
#2578=ORIENTED_EDGE('',*,*,#2026,.T.);
#2579=ORIENTED_EDGE('',*,*,#2027,.T.);
#2580=ORIENTED_EDGE('',*,*,#2028,.T.);
#2581=ORIENTED_EDGE('',*,*,#2029,.T.);
#2582=ORIENTED_EDGE('',*,*,#2026,.F.);
#2583=ORIENTED_EDGE('',*,*,#2029,.F.);
#2584=ORIENTED_EDGE('',*,*,#2027,.F.);
#2585=ORIENTED_EDGE('',*,*,#2028,.F.);
#2586=ORIENTED_EDGE('',*,*,#2030,.T.);
#2587=ORIENTED_EDGE('',*,*,#2031,.T.);
#2588=ORIENTED_EDGE('',*,*,#2030,.F.);
#2589=ORIENTED_EDGE('',*,*,#2031,.F.);
#2590=ORIENTED_EDGE('',*,*,#2032,.T.);
#2591=ORIENTED_EDGE('',*,*,#2032,.F.);
#2592=ORIENTED_EDGE('',*,*,#2033,.T.);
#2593=ORIENTED_EDGE('',*,*,#2034,.T.);
#2594=ORIENTED_EDGE('',*,*,#2033,.F.);
#2595=ORIENTED_EDGE('',*,*,#2035,.T.);
#2596=ORIENTED_EDGE('',*,*,#2034,.F.);
#2597=ORIENTED_EDGE('',*,*,#2036,.F.);
#2598=ORIENTED_EDGE('',*,*,#2037,.F.);
#2599=ORIENTED_EDGE('',*,*,#2038,.F.);
#2600=ORIENTED_EDGE('',*,*,#2039,.F.);
#2601=ORIENTED_EDGE('',*,*,#2035,.F.);
#2602=ORIENTED_EDGE('',*,*,#2040,.T.);
#2603=ORIENTED_EDGE('',*,*,#2041,.T.);
#2604=ORIENTED_EDGE('',*,*,#2042,.T.);
#2605=ORIENTED_EDGE('',*,*,#2040,.F.);
#2606=ORIENTED_EDGE('',*,*,#2043,.T.);
#2607=ORIENTED_EDGE('',*,*,#2044,.T.);
#2608=ORIENTED_EDGE('',*,*,#2045,.T.);
#2609=ORIENTED_EDGE('',*,*,#2046,.T.);
#2610=ORIENTED_EDGE('',*,*,#2047,.T.);
#2611=ORIENTED_EDGE('',*,*,#2048,.T.);
#2612=ORIENTED_EDGE('',*,*,#2048,.F.);
#2613=ORIENTED_EDGE('',*,*,#2049,.T.);
#2614=ORIENTED_EDGE('',*,*,#2050,.T.);
#2615=ORIENTED_EDGE('',*,*,#2051,.T.);
#2616=ORIENTED_EDGE('',*,*,#2049,.F.);
#2617=ORIENTED_EDGE('',*,*,#2050,.F.);
#2618=ORIENTED_EDGE('',*,*,#2051,.F.);
#2619=ORIENTED_EDGE('',*,*,#2052,.T.);
#2620=ORIENTED_EDGE('',*,*,#2053,.T.);
#2621=ORIENTED_EDGE('',*,*,#2052,.F.);
#2622=ORIENTED_EDGE('',*,*,#2054,.T.);
#2623=ORIENTED_EDGE('',*,*,#2053,.F.);
#2624=ORIENTED_EDGE('',*,*,#2054,.F.);
#2625=ORIENTED_EDGE('',*,*,#2055,.T.);
#2626=ORIENTED_EDGE('',*,*,#2056,.T.);
#2627=ORIENTED_EDGE('',*,*,#2057,.T.);
#2628=ORIENTED_EDGE('',*,*,#2008,.F.);
#2629=ORIENTED_EDGE('',*,*,#2058,.T.);
#2630=ORIENTED_EDGE('',*,*,#2055,.F.);
#2631=ORIENTED_EDGE('',*,*,#2009,.F.);
#2632=ORIENTED_EDGE('',*,*,#2057,.F.);
#2633=ORIENTED_EDGE('',*,*,#2059,.T.);
#2634=ORIENTED_EDGE('',*,*,#2010,.T.);
#2635=ORIENTED_EDGE('',*,*,#2011,.T.);
#2636=ORIENTED_EDGE('',*,*,#2059,.F.);
#2637=ORIENTED_EDGE('',*,*,#2056,.F.);
#2638=ORIENTED_EDGE('',*,*,#2058,.F.);
#2639=ORIENTED_EDGE('',*,*,#2007,.F.);
#2640=ORIENTED_EDGE('',*,*,#2002,.F.);
#2641=ORIENTED_EDGE('',*,*,#2060,.T.);
#2642=ORIENTED_EDGE('',*,*,#1997,.F.);
#2643=ORIENTED_EDGE('',*,*,#2061,.T.);
#2644=ORIENTED_EDGE('',*,*,#2062,.T.);
#2645=ORIENTED_EDGE('',*,*,#2061,.F.);
#2646=ORIENTED_EDGE('',*,*,#1996,.F.);
#2647=ORIENTED_EDGE('',*,*,#2063,.T.);
#2648=ORIENTED_EDGE('',*,*,#2062,.F.);
#2649=ORIENTED_EDGE('',*,*,#2064,.T.);
#2650=ORIENTED_EDGE('',*,*,#2065,.T.);
#2651=ORIENTED_EDGE('',*,*,#2066,.T.);
#2652=ORIENTED_EDGE('',*,*,#2067,.T.);
#2653=ORIENTED_EDGE('',*,*,#2068,.T.);
#2654=ORIENTED_EDGE('',*,*,#2069,.T.);
#2655=ORIENTED_EDGE('',*,*,#2070,.T.);
#2656=ORIENTED_EDGE('',*,*,#2071,.T.);
#2657=ORIENTED_EDGE('',*,*,#2072,.T.);
#2658=ORIENTED_EDGE('',*,*,#2071,.F.);
#2659=ORIENTED_EDGE('',*,*,#2073,.T.);
#2660=ORIENTED_EDGE('',*,*,#2072,.F.);
#2661=ORIENTED_EDGE('',*,*,#2073,.F.);
#2662=ORIENTED_EDGE('',*,*,#2074,.T.);
#2663=ORIENTED_EDGE('',*,*,#2075,.T.);
#2664=ORIENTED_EDGE('',*,*,#2074,.F.);
#2665=ORIENTED_EDGE('',*,*,#2076,.T.);
#2666=ORIENTED_EDGE('',*,*,#2077,.T.);
#2667=ORIENTED_EDGE('',*,*,#2075,.F.);
#2668=ORIENTED_EDGE('',*,*,#2078,.T.);
#2669=ORIENTED_EDGE('',*,*,#2078,.F.);
#2670=ORIENTED_EDGE('',*,*,#2079,.T.);
#2671=ORIENTED_EDGE('',*,*,#2025,.T.);
#2672=ORIENTED_EDGE('',*,*,#2079,.F.);
#2673=ORIENTED_EDGE('',*,*,#2080,.F.);
#2674=ORIENTED_EDGE('',*,*,#2081,.T.);
#2675=ORIENTED_EDGE('',*,*,#2082,.T.);
#2676=ORIENTED_EDGE('',*,*,#2081,.F.);
#2677=ORIENTED_EDGE('',*,*,#2082,.F.);
#2678=ORIENTED_EDGE('',*,*,#2083,.F.);
#2679=ORIENTED_EDGE('',*,*,#2084,.F.);
#2680=ORIENTED_EDGE('',*,*,#2085,.F.);
#2681=ORIENTED_EDGE('',*,*,#2086,.F.);
#2682=ORIENTED_EDGE('',*,*,#2005,.F.);
#2683=ORIENTED_EDGE('',*,*,#2080,.T.);
#2684=ORIENTED_EDGE('',*,*,#2087,.F.);
#2685=ORIENTED_EDGE('',*,*,#2088,.F.);
#2686=ORIENTED_EDGE('',*,*,#2089,.F.);
#2687=ORIENTED_EDGE('',*,*,#2090,.F.);
#2688=ORIENTED_EDGE('',*,*,#2091,.F.);
#2689=ORIENTED_EDGE('',*,*,#1999,.F.);
#2690=ORIENTED_EDGE('',*,*,#2092,.T.);
#2691=ORIENTED_EDGE('',*,*,#2015,.F.);
#2692=ORIENTED_EDGE('',*,*,#2093,.F.);
#2693=ORIENTED_EDGE('',*,*,#2019,.T.);
#2694=ORIENTED_EDGE('',*,*,#2094,.T.);
#2695=ORIENTED_EDGE('',*,*,#2000,.F.);
#2696=ORIENTED_EDGE('',*,*,#2093,.T.);
#2697=ORIENTED_EDGE('',*,*,#2014,.F.);
#2698=ORIENTED_EDGE('',*,*,#2006,.F.);
#2699=ORIENTED_EDGE('',*,*,#2095,.T.);
#2700=ORIENTED_EDGE('',*,*,#2020,.T.);
#2701=ORIENTED_EDGE('',*,*,#2016,.F.);
#2702=ORIENTED_EDGE('',*,*,#2092,.F.);
#2703=ORIENTED_EDGE('',*,*,#2076,.F.);
#2704=ORIENTED_EDGE('',*,*,#2077,.F.);
#2705=ORIENTED_EDGE('',*,*,#2096,.T.);
#2706=ORIENTED_EDGE('',*,*,#2091,.T.);
#2707=ORIENTED_EDGE('',*,*,#2096,.F.);
#2708=ORIENTED_EDGE('',*,*,#2086,.T.);
#2709=ORIENTED_EDGE('',*,*,#2097,.T.);
#2710=ORIENTED_EDGE('',*,*,#2090,.T.);
#2711=ORIENTED_EDGE('',*,*,#2097,.F.);
#2712=ORIENTED_EDGE('',*,*,#2085,.T.);
#2713=ORIENTED_EDGE('',*,*,#2098,.T.);
#2714=ORIENTED_EDGE('',*,*,#2089,.T.);
#2715=ORIENTED_EDGE('',*,*,#2098,.F.);
#2716=ORIENTED_EDGE('',*,*,#2084,.T.);
#2717=ORIENTED_EDGE('',*,*,#2099,.T.);
#2718=ORIENTED_EDGE('',*,*,#2088,.T.);
#2719=ORIENTED_EDGE('',*,*,#2099,.F.);
#2720=ORIENTED_EDGE('',*,*,#2083,.T.);
#2721=ORIENTED_EDGE('',*,*,#2100,.T.);
#2722=ORIENTED_EDGE('',*,*,#2087,.T.);
#2723=ORIENTED_EDGE('',*,*,#2100,.F.);
#2724=ORIENTED_EDGE('',*,*,#2047,.F.);
#2725=ORIENTED_EDGE('',*,*,#2101,.T.);
#2726=ORIENTED_EDGE('',*,*,#2039,.T.);
#2727=ORIENTED_EDGE('',*,*,#2101,.F.);
#2728=ORIENTED_EDGE('',*,*,#2046,.F.);
#2729=ORIENTED_EDGE('',*,*,#2102,.T.);
#2730=ORIENTED_EDGE('',*,*,#2038,.T.);
#2731=ORIENTED_EDGE('',*,*,#2102,.F.);
#2732=ORIENTED_EDGE('',*,*,#2045,.F.);
#2733=ORIENTED_EDGE('',*,*,#2103,.T.);
#2734=ORIENTED_EDGE('',*,*,#2037,.T.);
#2735=ORIENTED_EDGE('',*,*,#2103,.F.);
#2736=ORIENTED_EDGE('',*,*,#2044,.F.);
#2737=ORIENTED_EDGE('',*,*,#2104,.T.);
#2738=ORIENTED_EDGE('',*,*,#2036,.T.);
#2739=ORIENTED_EDGE('',*,*,#2104,.F.);
#2740=ORIENTED_EDGE('',*,*,#2068,.F.);
#2741=ORIENTED_EDGE('',*,*,#2105,.T.);
#2742=ORIENTED_EDGE('',*,*,#2106,.T.);
#2743=ORIENTED_EDGE('',*,*,#2107,.T.);
#2744=ORIENTED_EDGE('',*,*,#2105,.F.);
#2745=ORIENTED_EDGE('',*,*,#2108,.T.);
#2746=ORIENTED_EDGE('',*,*,#2106,.F.);
#2747=ORIENTED_EDGE('',*,*,#2107,.F.);
#2748=ORIENTED_EDGE('',*,*,#2108,.F.);
#2749=ORIENTED_EDGE('',*,*,#2067,.F.);
#2750=ORIENTED_EDGE('',*,*,#2109,.T.);
#2751=ORIENTED_EDGE('',*,*,#2024,.T.);
#2752=ORIENTED_EDGE('',*,*,#2109,.F.);
#2753=ORIENTED_EDGE('',*,*,#2066,.F.);
#2754=ORIENTED_EDGE('',*,*,#2110,.T.);
#2755=ORIENTED_EDGE('',*,*,#2023,.T.);
#2756=ORIENTED_EDGE('',*,*,#2110,.F.);
#2757=ORIENTED_EDGE('',*,*,#2065,.F.);
#2758=ORIENTED_EDGE('',*,*,#2111,.T.);
#2759=ORIENTED_EDGE('',*,*,#2022,.T.);
#2760=ORIENTED_EDGE('',*,*,#2111,.F.);
#2761=ORIENTED_EDGE('',*,*,#2001,.F.);
#2762=ORIENTED_EDGE('',*,*,#2094,.F.);
#2763=ORIENTED_EDGE('',*,*,#2018,.F.);
#2764=ORIENTED_EDGE('',*,*,#1998,.F.);
#2765=ORIENTED_EDGE('',*,*,#2060,.F.);
#2766=ORIENTED_EDGE('',*,*,#2003,.F.);
#2767=ORIENTED_EDGE('',*,*,#2063,.F.);
#2768=ORIENTED_EDGE('',*,*,#1995,.F.);
#2769=ORIENTED_EDGE('',*,*,#2021,.F.);
#2770=ORIENTED_EDGE('',*,*,#2095,.F.);
#2771=ORIENTED_EDGE('',*,*,#2069,.F.);
#2772=ORIENTED_EDGE('',*,*,#2070,.F.);
#2773=ORIENTED_EDGE('',*,*,#2112,.T.);
#2774=ORIENTED_EDGE('',*,*,#2064,.F.);
#2775=ORIENTED_EDGE('',*,*,#2112,.F.);
#2776=ORIENTED_EDGE('',*,*,#2043,.F.);
#2777=ORIENTED_EDGE('',*,*,#2113,.T.);
#2778=ORIENTED_EDGE('',*,*,#2041,.F.);
#2779=ORIENTED_EDGE('',*,*,#2042,.F.);
#2780=ORIENTED_EDGE('',*,*,#2113,.F.);
#3635=TOROIDAL_SURFACE('',#4016,88.0000000000002,2.);
#3636=TOROIDAL_SURFACE('',#4022,58.0000000000002,2.);
#3637=TOROIDAL_SURFACE('',#4065,41.9999999999999,2.);
#3638=TOROIDAL_SURFACE('',#4070,48.,8.);
#3639=TOROIDAL_SURFACE('',#4094,38.5,2.5);
#3640=TOROIDAL_SURFACE('',#4131,40.999999999998,1.);
#3641=TOROIDAL_SURFACE('',#4133,82.9999999999998,1.);
#3658=ADVANCED_FACE('',(#810),#3635,.T.);
#3659=ADVANCED_FACE('',(#811),#753,.T.);
#3660=ADVANCED_FACE('',(#812),#3636,.F.);
#3661=ADVANCED_FACE('',(#813,#195,#196,#197),#268,.T.);
#3662=ADVANCED_FACE('',(#814,#198),#269,.T.);
#3663=ADVANCED_FACE('',(#815),#163,.F.);
#3664=ADVANCED_FACE('',(#816),#754,.F.);
#3665=ADVANCED_FACE('',(#817,#199),#270,.T.);
#3666=ADVANCED_FACE('',(#818),#755,.F.);
#3667=ADVANCED_FACE('',(#819,#200,#201,#202,#203,#204),#271,.T.);
#3668=ADVANCED_FACE('',(#820),#756,.T.);
#3669=ADVANCED_FACE('',(#821,#205,#206,#207,#208,#209),#272,.T.);
#3670=ADVANCED_FACE('',(#822),#757,.T.);
#3671=ADVANCED_FACE('',(#823),#3637,.F.);
#3672=ADVANCED_FACE('',(#824,#210),#273,.T.);
#3673=ADVANCED_FACE('',(#825),#3638,.T.);
#3674=ADVANCED_FACE('',(#826),#758,.T.);
#3675=ADVANCED_FACE('',(#827),#759,.T.);
#3676=ADVANCED_FACE('',(#828,#211,#212,#213,#214,#215),#274,.T.);
#3677=ADVANCED_FACE('',(#829),#760,.F.);
#3678=ADVANCED_FACE('',(#830,#216),#275,.T.);
#3679=ADVANCED_FACE('',(#831,#217),#761,.F.);
#3680=ADVANCED_FACE('',(#832,#218),#276,.T.);
#3681=ADVANCED_FACE('',(#833),#3639,.F.);
#3682=ADVANCED_FACE('',(#834),#762,.T.);
#3683=ADVANCED_FACE('',(#835,#219,#220,#221,#222,#223),#277,.F.);
#3684=ADVANCED_FACE('',(#836,#224,#225,#226,#227,#228),#278,.T.);
#3685=ADVANCED_FACE('',(#837),#763,.F.);
#3686=ADVANCED_FACE('',(#838),#279,.F.);
#3687=ADVANCED_FACE('',(#839),#280,.F.);
#3688=ADVANCED_FACE('',(#840),#764,.F.);
#3689=ADVANCED_FACE('',(#841),#765,.F.);
#3690=ADVANCED_FACE('',(#842),#766,.F.);
#3691=ADVANCED_FACE('',(#843),#767,.F.);
#3692=ADVANCED_FACE('',(#844),#768,.F.);
#3693=ADVANCED_FACE('',(#845),#769,.F.);
#3694=ADVANCED_FACE('',(#846),#770,.F.);
#3695=ADVANCED_FACE('',(#847),#771,.F.);
#3696=ADVANCED_FACE('',(#848),#772,.F.);
#3697=ADVANCED_FACE('',(#849),#773,.F.);
#3698=ADVANCED_FACE('',(#850),#164,.F.);
#3699=ADVANCED_FACE('',(#851),#774,.F.);
#3700=ADVANCED_FACE('',(#852),#775,.F.);
#3701=ADVANCED_FACE('',(#853),#776,.F.);
#3702=ADVANCED_FACE('',(#854),#777,.T.);
#3703=ADVANCED_FACE('',(#855),#778,.T.);
#3704=ADVANCED_FACE('',(#856),#3640,.T.);
#3705=ADVANCED_FACE('',(#857),#3641,.T.);
#3881=CLOSED_SHELL('',(#3658,#3659,#3660,#3661,#3662,#3663,#3664,#3665,
#3666,#3667,#3668,#3669,#3670,#3671,#3672,#3673,#3674,#3675,#3676,#3677,
#3678,#3679,#3680,#3681,#3682,#3683,#3684,#3685,#3686,#3687,#3688,#3689,
#3690,#3691,#3692,#3693,#3694,#3695,#3696,#3697,#3698,#3699,#3700,#3701,
#3702,#3703,#3704,#3705));
#4015=AXIS2_PLACEMENT_3D('',#5571,#4471,#4472);
#4016=AXIS2_PLACEMENT_3D('',#5572,#4473,#4474);
#4017=AXIS2_PLACEMENT_3D('',#5575,#4475,#4476);
#4018=AXIS2_PLACEMENT_3D('',#5586,#4477,#4478);
#4019=AXIS2_PLACEMENT_3D('',#5588,#4479,#4480);
#4020=AXIS2_PLACEMENT_3D('',#5599,#4481,#4482);
#4021=AXIS2_PLACEMENT_3D('',#5689,#4485,#4486);
#4022=AXIS2_PLACEMENT_3D('',#5775,#4488,#4489);
#4023=AXIS2_PLACEMENT_3D('',#5778,#4490,#4491);
#4024=AXIS2_PLACEMENT_3D('',#5779,#4492,#4493);
#4025=AXIS2_PLACEMENT_3D('',#5781,#4494,#4495);
#4026=AXIS2_PLACEMENT_3D('',#5783,#4496,#4497);
#4027=AXIS2_PLACEMENT_3D('',#5991,#4498,#4499);
#4028=AXIS2_PLACEMENT_3D('',#5992,#4500,#4501);
#4029=AXIS2_PLACEMENT_3D('',#5994,#4502,#4503);
#4030=AXIS2_PLACEMENT_3D('',#5998,#4506,#4507);
#4031=AXIS2_PLACEMENT_3D('',#6000,#4508,#4509);
#4032=AXIS2_PLACEMENT_3D('',#6002,#4510,#4511);
#4033=AXIS2_PLACEMENT_3D('',#6004,#4512,#4513);
#4034=AXIS2_PLACEMENT_3D('',#6005,#4514,#4515);
#4035=AXIS2_PLACEMENT_3D('',#6007,#4516,#4517);
#4036=AXIS2_PLACEMENT_3D('',#6009,#4518,#4519);
#4037=AXIS2_PLACEMENT_3D('',#6010,#4520,#4521);
#4038=AXIS2_PLACEMENT_3D('',#6013,#4522,#4523);
#4039=AXIS2_PLACEMENT_3D('',#6014,#4524,#4525);
#4040=AXIS2_PLACEMENT_3D('',#6016,#4527,#4528);
#4041=AXIS2_PLACEMENT_3D('',#6019,#4530,#4531);
#4042=AXIS2_PLACEMENT_3D('',#6020,#4532,#4533);
#4043=AXIS2_PLACEMENT_3D('',#6022,#4534,#4535);
#4044=AXIS2_PLACEMENT_3D('',#6023,#4536,#4537);
#4045=AXIS2_PLACEMENT_3D('',#6026,#4539,#4540);
#4046=AXIS2_PLACEMENT_3D('',#6027,#4541,#4542);
#4047=AXIS2_PLACEMENT_3D('',#6029,#4543,#4544);
#4048=AXIS2_PLACEMENT_3D('',#6031,#4545,#4546);
#4049=AXIS2_PLACEMENT_3D('',#6033,#4547,#4548);
#4050=AXIS2_PLACEMENT_3D('',#6035,#4549,#4550);
#4051=AXIS2_PLACEMENT_3D('',#6037,#4551,#4552);
#4052=AXIS2_PLACEMENT_3D('',#6038,#4553,#4554);
#4053=AXIS2_PLACEMENT_3D('',#6042,#4556,#4557);
#4054=AXIS2_PLACEMENT_3D('',#6043,#4558,#4559);
#4055=AXIS2_PLACEMENT_3D('',#6044,#4560,#4561);
#4056=AXIS2_PLACEMENT_3D('',#6046,#4562,#4563);
#4057=AXIS2_PLACEMENT_3D('',#6048,#4564,#4565);
#4058=AXIS2_PLACEMENT_3D('',#6050,#4566,#4567);
#4059=AXIS2_PLACEMENT_3D('',#6052,#4568,#4569);
#4060=AXIS2_PLACEMENT_3D('',#6054,#4570,#4571);
#4061=AXIS2_PLACEMENT_3D('',#6056,#4572,#4573);
#4062=AXIS2_PLACEMENT_3D('',#6057,#4574,#4575);
#4063=AXIS2_PLACEMENT_3D('',#6061,#4577,#4578);
#4064=AXIS2_PLACEMENT_3D('',#6062,#4579,#4580);
#4065=AXIS2_PLACEMENT_3D('',#6063,#4581,#4582);
#4066=AXIS2_PLACEMENT_3D('',#6065,#4583,#4584);
#4067=AXIS2_PLACEMENT_3D('',#6066,#4585,#4586);
#4068=AXIS2_PLACEMENT_3D('',#6067,#4587,#4588);
#4069=AXIS2_PLACEMENT_3D('',#6069,#4589,#4590);
#4070=AXIS2_PLACEMENT_3D('',#6070,#4591,#4592);
#4071=AXIS2_PLACEMENT_3D('',#6072,#4593,#4594);
#4072=AXIS2_PLACEMENT_3D('',#6074,#4595,#4596);
#4073=AXIS2_PLACEMENT_3D('',#6075,#4597,#4598);
#4074=AXIS2_PLACEMENT_3D('',#6076,#4599,#4600);
#4075=AXIS2_PLACEMENT_3D('',#6077,#4601,#4602);
#4076=AXIS2_PLACEMENT_3D('',#6079,#4604,#4605);
#4077=AXIS2_PLACEMENT_3D('',#6083,#4608,#4609);
#4078=AXIS2_PLACEMENT_3D('',#6085,#4611,#4612);
#4079=AXIS2_PLACEMENT_3D('',#6087,#4613,#4614);
#4080=AXIS2_PLACEMENT_3D('',#6089,#4615,#4616);
#4081=AXIS2_PLACEMENT_3D('',#6091,#4617,#4618);
#4082=AXIS2_PLACEMENT_3D('',#6093,#4619,#4620);
#4083=AXIS2_PLACEMENT_3D('',#6095,#4621,#4622);
#4084=AXIS2_PLACEMENT_3D('',#6096,#4623,#4624);
#4085=AXIS2_PLACEMENT_3D('',#6099,#4625,#4626);
#4086=AXIS2_PLACEMENT_3D('',#6100,#4627,#4628);
#4087=AXIS2_PLACEMENT_3D('',#6103,#4630,#4631);
#4088=AXIS2_PLACEMENT_3D('',#6104,#4632,#4633);
#4089=AXIS2_PLACEMENT_3D('',#6106,#4634,#4635);
#4090=AXIS2_PLACEMENT_3D('',#6107,#4636,#4637);
#4091=AXIS2_PLACEMENT_3D('',#6110,#4639,#4640);
#4092=AXIS2_PLACEMENT_3D('',#6181,#4641,#4642);
#4093=AXIS2_PLACEMENT_3D('',#6183,#4643,#4644);
#4094=AXIS2_PLACEMENT_3D('',#6184,#4645,#4646);
#4095=AXIS2_PLACEMENT_3D('',#6185,#4647,#4648);
#4096=AXIS2_PLACEMENT_3D('',#6186,#4649,#4650);
#4097=AXIS2_PLACEMENT_3D('',#6188,#4651,#4652);
#4098=AXIS2_PLACEMENT_3D('',#6191,#4654,#4655);
#4099=AXIS2_PLACEMENT_3D('',#6192,#4656,#4657);
#4100=AXIS2_PLACEMENT_3D('',#6194,#4658,#4659);
#4101=AXIS2_PLACEMENT_3D('',#6196,#4660,#4661);
#4102=AXIS2_PLACEMENT_3D('',#6198,#4662,#4663);
#4103=AXIS2_PLACEMENT_3D('',#6200,#4664,#4665);
#4104=AXIS2_PLACEMENT_3D('',#6201,#4666,#4667);
#4105=AXIS2_PLACEMENT_3D('',#6203,#4668,#4669);
#4106=AXIS2_PLACEMENT_3D('',#6205,#4670,#4671);
#4107=AXIS2_PLACEMENT_3D('',#6207,#4672,#4673);
#4108=AXIS2_PLACEMENT_3D('',#6209,#4674,#4675);
#4109=AXIS2_PLACEMENT_3D('',#6211,#4676,#4677);
#4110=AXIS2_PLACEMENT_3D('',#6212,#4678,#4679);
#4111=AXIS2_PLACEMENT_3D('',#6215,#4682,#4683);
#4112=AXIS2_PLACEMENT_3D('',#6217,#4685,#4686);
#4113=AXIS2_PLACEMENT_3D('',#6219,#4688,#4689);
#4114=AXIS2_PLACEMENT_3D('',#6221,#4691,#4692);
#4115=AXIS2_PLACEMENT_3D('',#6223,#4694,#4695);
#4116=AXIS2_PLACEMENT_3D('',#6225,#4697,#4698);
#4117=AXIS2_PLACEMENT_3D('',#6227,#4700,#4701);
#4118=AXIS2_PLACEMENT_3D('',#6229,#4703,#4704);
#4119=AXIS2_PLACEMENT_3D('',#6231,#4706,#4707);
#4120=AXIS2_PLACEMENT_3D('',#6233,#4709,#4710);
#4121=AXIS2_PLACEMENT_3D('',#6235,#4712,#4713);
#4122=AXIS2_PLACEMENT_3D('',#6237,#4715,#4716);
#4123=AXIS2_PLACEMENT_3D('',#6241,#4718,#4719);
#4124=AXIS2_PLACEMENT_3D('',#6242,#4720,#4721);
#4125=AXIS2_PLACEMENT_3D('',#6243,#4722,#4723);
#4126=AXIS2_PLACEMENT_3D('',#6246,#4725,#4726);
#4127=AXIS2_PLACEMENT_3D('',#6248,#4728,#4729);
#4128=AXIS2_PLACEMENT_3D('',#6250,#4731,#4732);
#4129=AXIS2_PLACEMENT_3D('',#6252,#4734,#4735);
#4130=AXIS2_PLACEMENT_3D('',#6253,#4736,#4737);
#4131=AXIS2_PLACEMENT_3D('',#6254,#4738,#4739);
#4132=AXIS2_PLACEMENT_3D('',#6255,#4740,#4741);
#4133=AXIS2_PLACEMENT_3D('',#6256,#4742,#4743);
#4134=AXIS2_PLACEMENT_3D('',#6257,#4744,#4745);
#4471=DIRECTION('axis',(0.,0.,1.));
#4472=DIRECTION('refdir',(1.,0.,0.));
#4473=DIRECTION('center_axis',(3.43024899888577E-15,-1.,0.));
#4474=DIRECTION('ref_axis',(-1.,-3.31586610021379E-15,-6.12323399573677E-17));
#4475=DIRECTION('center_axis',(3.43024899888577E-15,-1.,0.));
#4476=DIRECTION('ref_axis',(1.,3.43024899888577E-15,0.));
#4477=DIRECTION('center_axis',(3.43024899888577E-15,-1.,0.));
#4478=DIRECTION('ref_axis',(1.,3.43024899888577E-15,0.));
#4479=DIRECTION('center_axis',(3.43024899888577E-15,-1.,0.));
#4480=DIRECTION('ref_axis',(1.,3.43024899888577E-15,0.));
#4481=DIRECTION('center_axis',(1.,0.,0.));
#4482=DIRECTION('ref_axis',(0.,0.,-1.));
#4483=DIRECTION('',(1.,3.39178734177461E-15,0.));
#4484=DIRECTION('',(-1.,0.,0.));
#4485=DIRECTION('center_axis',(1.,0.,0.));
#4486=DIRECTION('ref_axis',(0.,0.,-1.));
#4487=DIRECTION('',(-1.,-3.39178430813906E-15,0.));
#4488=DIRECTION('center_axis',(3.43024899888577E-15,-1.,0.));
#4489=DIRECTION('ref_axis',(0.,0.,-1.));
#4490=DIRECTION('center_axis',(3.43024899888577E-15,-1.,0.));
#4491=DIRECTION('ref_axis',(1.,3.43024899888577E-15,0.));
#4492=DIRECTION('center_axis',(3.43024899888577E-15,-1.,0.));
#4493=DIRECTION('ref_axis',(1.,3.43024899888577E-15,0.));
#4494=DIRECTION('center_axis',(1.,3.43024899888577E-15,1.22464679914735E-16));
#4495=DIRECTION('ref_axis',(-1.22464679914735E-16,0.,1.));
#4496=DIRECTION('center_axis',(3.43024899888577E-15,-1.,0.));
#4497=DIRECTION('ref_axis',(1.,3.43024899888577E-15,0.));
#4498=DIRECTION('center_axis',(3.43024899888577E-15,-1.,0.));
#4499=DIRECTION('ref_axis',(1.,3.43024899888577E-15,0.));
#4500=DIRECTION('center_axis',(3.43024899888577E-15,-1.,0.));
#4501=DIRECTION('ref_axis',(0.,0.,-1.));
#4502=DIRECTION('center_axis',(3.43024899888577E-15,-1.,0.));
#4503=DIRECTION('ref_axis',(1.,3.43024899888577E-15,0.));
#4504=DIRECTION('',(1.,3.40592503341502E-15,0.));
#4505=DIRECTION('',(-1.,-3.40592503341502E-15,0.));
#4506=DIRECTION('center_axis',(3.43024899888577E-15,-1.,0.));
#4507=DIRECTION('ref_axis',(1.,3.43024899888577E-15,0.));
#4508=DIRECTION('center_axis',(3.43024899888577E-15,-1.,0.));
#4509=DIRECTION('ref_axis',(1.,3.43024899888577E-15,0.));
#4510=DIRECTION('center_axis',(3.43024899888577E-15,-1.,0.));
#4511=DIRECTION('ref_axis',(1.,3.43024899888577E-15,0.));
#4512=DIRECTION('center_axis',(3.43024899888577E-15,-1.,0.));
#4513=DIRECTION('ref_axis',(1.,3.43024899888577E-15,0.));
#4514=DIRECTION('center_axis',(-3.43024899888577E-15,1.,0.));
#4515=DIRECTION('ref_axis',(0.,0.,1.));
#4516=DIRECTION('center_axis',(3.43024899888577E-15,-1.,0.));
#4517=DIRECTION('ref_axis',(1.,3.43024899888577E-15,0.));
#4518=DIRECTION('center_axis',(3.43024899888577E-15,-1.,0.));
#4519=DIRECTION('ref_axis',(1.,3.43024899888577E-15,0.));
#4520=DIRECTION('center_axis',(-3.43024899888577E-15,1.,0.));
#4521=DIRECTION('ref_axis',(-1.,-3.43024899888577E-15,0.));
#4522=DIRECTION('center_axis',(3.43024899888577E-15,-1.,0.));
#4523=DIRECTION('ref_axis',(1.,3.43024899888577E-15,0.));
#4524=DIRECTION('center_axis',(3.43024899888577E-15,-1.,0.));
#4525=DIRECTION('ref_axis',(1.,3.43024899888577E-15,0.));
#4526=DIRECTION('',(0.707106781186544,0.707106781186551,-8.65956056235492E-17));
#4527=DIRECTION('center_axis',(3.43024899888577E-15,-1.,0.));
#4528=DIRECTION('ref_axis',(1.,3.43024899888577E-15,0.));
#4529=DIRECTION('',(3.43024899888577E-15,-1.,0.));
#4530=DIRECTION('center_axis',(3.43024899888577E-15,-1.,0.));
#4531=DIRECTION('ref_axis',(1.,3.43024899888577E-15,0.));
#4532=DIRECTION('center_axis',(-3.43024899888577E-15,1.,0.));
#4533=DIRECTION('ref_axis',(0.,0.,1.));
#4534=DIRECTION('center_axis',(3.43024899888577E-15,-1.,0.));
#4535=DIRECTION('ref_axis',(1.,3.43024899888577E-15,0.));
#4536=DIRECTION('center_axis',(3.43024899888577E-15,-1.,0.));
#4537=DIRECTION('ref_axis',(1.,3.43024899888577E-15,0.));
#4538=DIRECTION('',(3.43024899888577E-15,-1.,0.));
#4539=DIRECTION('center_axis',(3.43024899888577E-15,-1.,0.));
#4540=DIRECTION('ref_axis',(1.,3.43024899888577E-15,0.));
#4541=DIRECTION('center_axis',(3.43024899888577E-15,-1.,0.));
#4542=DIRECTION('ref_axis',(0.,0.,-1.));
#4543=DIRECTION('center_axis',(3.43024899888577E-15,-1.,0.));
#4544=DIRECTION('ref_axis',(1.,3.43024899888577E-15,0.));
#4545=DIRECTION('center_axis',(3.43024899888577E-15,-1.,0.));
#4546=DIRECTION('ref_axis',(-3.49148133884313E-15,-1.22273440309257E-29,
-1.));
#4547=DIRECTION('center_axis',(3.43024899888577E-15,-1.,0.));
#4548=DIRECTION('ref_axis',(-1.,-3.43024899888577E-15,0.));
#4549=DIRECTION('center_axis',(3.43024899888577E-15,-1.,0.));
#4550=DIRECTION('ref_axis',(1.04744440165294E-14,3.5893171187556E-29,1.));
#4551=DIRECTION('center_axis',(3.43024899888577E-15,-1.,0.));
#4552=DIRECTION('ref_axis',(1.,3.43024899888577E-15,0.));
#4553=DIRECTION('center_axis',(3.43024899888577E-15,-1.,0.));
#4554=DIRECTION('ref_axis',(1.,3.43024899888577E-15,0.));
#4555=DIRECTION('',(-3.43024899888577E-15,1.,0.));
#4556=DIRECTION('center_axis',(-3.43024899888577E-15,1.,0.));
#4557=DIRECTION('ref_axis',(-1.,-3.43024899888577E-15,0.));
#4558=DIRECTION('center_axis',(-3.43024899888577E-15,1.,0.));
#4559=DIRECTION('ref_axis',(-1.,-3.43024899888577E-15,0.));
#4560=DIRECTION('center_axis',(-3.43024899888577E-15,1.,0.));
#4561=DIRECTION('ref_axis',(0.,0.,1.));
#4562=DIRECTION('center_axis',(-3.43024899888577E-15,1.,0.));
#4563=DIRECTION('ref_axis',(-1.,-3.43024899888577E-15,0.));
#4564=DIRECTION('center_axis',(-3.43024899888577E-15,1.,0.));
#4565=DIRECTION('ref_axis',(-1.,-3.43024899888577E-15,0.));
#4566=DIRECTION('center_axis',(-3.43024899888577E-15,1.,0.));
#4567=DIRECTION('ref_axis',(-1.,-3.43024899888577E-15,0.));
#4568=DIRECTION('center_axis',(-3.43024899888577E-15,1.,0.));
#4569=DIRECTION('ref_axis',(-1.,-3.43024899888577E-15,0.));
#4570=DIRECTION('center_axis',(-3.43024899888577E-15,1.,0.));
#4571=DIRECTION('ref_axis',(-1.,-3.43024899888577E-15,0.));
#4572=DIRECTION('center_axis',(3.43024899888577E-15,-1.,0.));
#4573=DIRECTION('ref_axis',(1.,3.43024899888577E-15,0.));
#4574=DIRECTION('center_axis',(3.43024899888577E-15,-1.,0.));
#4575=DIRECTION('ref_axis',(1.,3.43024899888577E-15,0.));
#4576=DIRECTION('',(-3.43024899888577E-15,1.,0.));
#4577=DIRECTION('center_axis',(3.43024899888577E-15,-1.,0.));
#4578=DIRECTION('ref_axis',(1.,3.43024899888577E-15,0.));
#4579=DIRECTION('center_axis',(3.43024899888577E-15,-1.,0.));
#4580=DIRECTION('ref_axis',(1.,3.43024899888577E-15,0.));
#4581=DIRECTION('center_axis',(3.43024899888577E-15,-1.,0.));
#4582=DIRECTION('ref_axis',(0.,0.,-1.));
#4583=DIRECTION('center_axis',(1.,3.43024899888577E-15,1.22464679914735E-16));
#4584=DIRECTION('ref_axis',(-1.22464679914735E-16,0.,1.));
#4585=DIRECTION('center_axis',(3.43024899888577E-15,-1.,0.));
#4586=DIRECTION('ref_axis',(1.,3.43024899888577E-15,0.));
#4587=DIRECTION('center_axis',(3.43024899888577E-15,-1.,0.));
#4588=DIRECTION('ref_axis',(0.,0.,-1.));
#4589=DIRECTION('center_axis',(3.43024899888577E-15,-1.,0.));
#4590=DIRECTION('ref_axis',(1.,3.43024899888577E-15,0.));
#4591=DIRECTION('center_axis',(3.43024899888577E-15,-1.,0.));
#4592=DIRECTION('ref_axis',(0.,0.,-1.));
#4593=DIRECTION('center_axis',(-1.,-3.43024899888577E-15,-1.22464679914735E-16));
#4594=DIRECTION('ref_axis',(-1.22464679914735E-16,0.,1.));
#4595=DIRECTION('center_axis',(3.43024899888577E-15,-1.,0.));
#4596=DIRECTION('ref_axis',(1.,3.43024899888577E-15,0.));
#4597=DIRECTION('center_axis',(3.43024899888577E-15,-1.,0.));
#4598=DIRECTION('ref_axis',(1.,3.43024899888577E-15,0.));
#4599=DIRECTION('center_axis',(3.43024899888577E-15,-1.,0.));
#4600=DIRECTION('ref_axis',(1.,3.43024899888577E-15,0.));
#4601=DIRECTION('center_axis',(3.43024899888577E-15,-1.,0.));
#4602=DIRECTION('ref_axis',(1.,3.43024899888577E-15,0.));
#4603=DIRECTION('',(-3.43024899888577E-15,1.,0.));
#4604=DIRECTION('center_axis',(3.43024899888577E-15,-1.,0.));
#4605=DIRECTION('ref_axis',(1.,3.43024899888577E-15,0.));
#4606=DIRECTION('',(2.23596159769488E-15,-1.,0.));
#4607=DIRECTION('',(-3.43024899888577E-15,1.,0.));
#4608=DIRECTION('center_axis',(3.43024899888577E-15,-1.,0.));
#4609=DIRECTION('ref_axis',(1.,3.43024899888577E-15,0.));
#4610=DIRECTION('',(2.23596159769488E-15,-1.,0.));
#4611=DIRECTION('center_axis',(-3.43024899888577E-15,1.,0.));
#4612=DIRECTION('ref_axis',(0.,0.,1.));
#4613=DIRECTION('center_axis',(-3.43024899888577E-15,1.,0.));
#4614=DIRECTION('ref_axis',(-1.,-3.43024899888577E-15,0.));
#4615=DIRECTION('center_axis',(3.43024899888572E-15,-1.,-3.43024899888575E-15));
#4616=DIRECTION('ref_axis',(1.,3.43024899888575E-15,-1.04744440165294E-14));
#4617=DIRECTION('center_axis',(6.86049799777151E-15,-1.,0.));
#4618=DIRECTION('ref_axis',(0.,0.,1.));
#4619=DIRECTION('center_axis',(3.43024899888577E-15,-1.,3.43024899888575E-15));
#4620=DIRECTION('ref_axis',(-1.,-3.43024899888575E-15,3.49148133884313E-15));
#4621=DIRECTION('center_axis',(0.,-1.,0.));
#4622=DIRECTION('ref_axis',(0.,0.,-1.));
#4623=DIRECTION('center_axis',(3.43024899888577E-15,-1.,0.));
#4624=DIRECTION('ref_axis',(1.,3.43024899888577E-15,0.));
#4625=DIRECTION('center_axis',(-3.43024899888577E-15,1.,0.));
#4626=DIRECTION('ref_axis',(-1.,-3.43024899888577E-15,0.));
#4627=DIRECTION('center_axis',(-3.43024899888577E-15,1.,0.));
#4628=DIRECTION('ref_axis',(-1.,-3.43024899888577E-15,0.));
#4629=DIRECTION('',(3.43024899888577E-15,-1.,0.));
#4630=DIRECTION('center_axis',(3.43024899888577E-15,-1.,0.));
#4631=DIRECTION('ref_axis',(1.,3.43024899888577E-15,0.));
#4632=DIRECTION('center_axis',(3.43024899888577E-15,-1.,0.));
#4633=DIRECTION('ref_axis',(0.,0.,-1.));
#4634=DIRECTION('center_axis',(3.43024899888577E-15,-1.,0.));
#4635=DIRECTION('ref_axis',(1.,3.43024899888577E-15,0.));
#4636=DIRECTION('center_axis',(3.43024899888577E-15,-1.,0.));
#4637=DIRECTION('ref_axis',(1.,3.43024899888577E-15,0.));
#4638=DIRECTION('',(3.43024899888577E-15,-1.,0.));
#4639=DIRECTION('center_axis',(3.43024899888577E-15,-1.,0.));
#4640=DIRECTION('ref_axis',(1.,3.43024899888577E-15,0.));
#4641=DIRECTION('center_axis',(-3.43024899888577E-15,1.,0.));
#4642=DIRECTION('ref_axis',(0.,0.,1.));
#4643=DIRECTION('center_axis',(3.43024899888577E-15,-1.,0.));
#4644=DIRECTION('ref_axis',(1.,3.43024899888577E-15,0.));
#4645=DIRECTION('center_axis',(3.43024899888577E-15,-1.,0.));
#4646=DIRECTION('ref_axis',(0.,0.,-1.));
#4647=DIRECTION('center_axis',(1.,3.43024899888577E-15,1.22464679914735E-16));
#4648=DIRECTION('ref_axis',(-1.22464679914735E-16,-3.84810197668786E-31,
1.));
#4649=DIRECTION('center_axis',(1.,0.,0.));
#4650=DIRECTION('ref_axis',(0.,0.,-1.));
#4651=DIRECTION('center_axis',(1.,0.,0.));
#4652=DIRECTION('ref_axis',(0.,0.,-1.));
#4653=DIRECTION('',(-1.,0.,0.));
#4654=DIRECTION('center_axis',(1.,0.,0.));
#4655=DIRECTION('ref_axis',(0.,0.,-1.));
#4656=DIRECTION('center_axis',(1.,0.,0.));
#4657=DIRECTION('ref_axis',(0.,0.,-1.));
#4658=DIRECTION('center_axis',(1.,0.,0.));
#4659=DIRECTION('ref_axis',(0.,0.,-1.));
#4660=DIRECTION('center_axis',(1.,0.,0.));
#4661=DIRECTION('ref_axis',(0.,0.,-1.));
#4662=DIRECTION('center_axis',(1.,0.,0.));
#4663=DIRECTION('ref_axis',(0.,0.,-1.));
#4664=DIRECTION('center_axis',(1.,0.,0.));
#4665=DIRECTION('ref_axis',(0.,0.,-1.));
#4666=DIRECTION('center_axis',(1.,0.,0.));
#4667=DIRECTION('ref_axis',(0.,0.,-1.));
#4668=DIRECTION('center_axis',(1.,0.,0.));
#4669=DIRECTION('ref_axis',(0.,-1.,3.49148133884313E-15));
#4670=DIRECTION('center_axis',(1.,0.,0.));
#4671=DIRECTION('ref_axis',(0.,0.,1.));
#4672=DIRECTION('center_axis',(1.,0.,0.));
#4673=DIRECTION('ref_axis',(0.,1.,-1.04744440165294E-14));
#4674=DIRECTION('center_axis',(1.,0.,0.));
#4675=DIRECTION('ref_axis',(0.,0.,-1.));
#4676=DIRECTION('center_axis',(1.,0.,0.));
#4677=DIRECTION('ref_axis',(0.,0.,-1.));
#4678=DIRECTION('center_axis',(-3.43024899888577E-15,1.,0.));
#4679=DIRECTION('ref_axis',(0.999999999999977,3.43024899888569E-15,2.15720406748434E-7));
#4680=DIRECTION('',(-3.55190708269137E-15,1.,0.));
#4681=DIRECTION('',(-3.32971747973986E-15,1.,0.));
#4682=DIRECTION('center_axis',(0.,0.,1.));
#4683=DIRECTION('ref_axis',(1.,0.,0.));
#4684=DIRECTION('',(-3.38353683695286E-15,1.,0.));
#4685=DIRECTION('center_axis',(0.,0.,-1.));
#4686=DIRECTION('ref_axis',(-1.,0.,0.));
#4687=DIRECTION('',(-3.38353683695286E-15,1.,0.));
#4688=DIRECTION('center_axis',(1.,0.,0.));
#4689=DIRECTION('ref_axis',(0.,0.,-1.));
#4690=DIRECTION('',(1.,0.,0.));
#4691=DIRECTION('center_axis',(1.,0.,0.));
#4692=DIRECTION('ref_axis',(0.,0.,-1.));
#4693=DIRECTION('',(1.,0.,0.));
#4694=DIRECTION('center_axis',(1.,0.,0.));
#4695=DIRECTION('ref_axis',(0.,0.,-1.));
#4696=DIRECTION('',(1.,0.,0.));
#4697=DIRECTION('center_axis',(1.,0.,0.));
#4698=DIRECTION('ref_axis',(0.,0.,-1.));
#4699=DIRECTION('',(1.,0.,0.));
#4700=DIRECTION('center_axis',(1.,0.,0.));
#4701=DIRECTION('ref_axis',(0.,0.,-1.));
#4702=DIRECTION('',(1.,0.,0.));
#4703=DIRECTION('center_axis',(3.43024899888577E-15,-1.,0.));
#4704=DIRECTION('ref_axis',(1.,3.43024899888577E-15,0.));
#4705=DIRECTION('',(3.43024899888577E-15,-1.,0.));
#4706=DIRECTION('center_axis',(3.43024899888577E-15,-1.,0.));
#4707=DIRECTION('ref_axis',(1.,3.43024899888577E-15,0.));
#4708=DIRECTION('',(3.43024899888577E-15,-1.,0.));
#4709=DIRECTION('center_axis',(3.43024899888577E-15,-1.,0.));
#4710=DIRECTION('ref_axis',(1.,3.43024899888577E-15,0.));
#4711=DIRECTION('',(3.43024899888577E-15,-1.,0.));
#4712=DIRECTION('center_axis',(3.43024899888577E-15,-1.,0.));
#4713=DIRECTION('ref_axis',(1.,3.43024899888577E-15,0.));
#4714=DIRECTION('',(3.43024899888577E-15,-1.,0.));
#4715=DIRECTION('center_axis',(0.,-1.,0.));
#4716=DIRECTION('ref_axis',(0.,0.,-1.));
#4717=DIRECTION('',(0.,-1.,0.));
#4718=DIRECTION('center_axis',(0.,-1.,0.));
#4719=DIRECTION('ref_axis',(0.,0.,-1.));
#4720=DIRECTION('center_axis',(0.,-1.,0.));
#4721=DIRECTION('ref_axis',(0.,0.,-1.));
#4722=DIRECTION('center_axis',(0.,1.,0.));
#4723=DIRECTION('ref_axis',(0.,0.,1.));
#4724=DIRECTION('',(-1.04972719113862E-16,0.515038074910052,-0.857167300702114));
#4725=DIRECTION('center_axis',(3.43024899888577E-15,-1.,3.43024899888575E-15));
#4726=DIRECTION('ref_axis',(-1.,-3.43024899888575E-15,3.49148133884313E-15));
#4727=DIRECTION('',(3.43024899888577E-15,-1.,3.43024899888575E-15));
#4728=DIRECTION('center_axis',(6.86049799777151E-15,-1.,0.));
#4729=DIRECTION('ref_axis',(0.,0.,1.));
#4730=DIRECTION('',(6.86049799777151E-15,-1.,0.));
#4731=DIRECTION('center_axis',(3.43024899888572E-15,-1.,-3.43024899888575E-15));
#4732=DIRECTION('ref_axis',(1.,3.43024899888575E-15,-1.04744440165294E-14));
#4733=DIRECTION('',(3.43024899888572E-15,-1.,-3.43024899888575E-15));
#4734=DIRECTION('center_axis',(3.43024899888577E-15,-1.,0.));
#4735=DIRECTION('ref_axis',(1.,3.43024899888577E-15,0.));
#4736=DIRECTION('center_axis',(3.43024899888577E-15,-1.,0.));
#4737=DIRECTION('ref_axis',(1.,3.43024899888577E-15,0.));
#4738=DIRECTION('center_axis',(-3.43024899888577E-15,1.,0.));
#4739=DIRECTION('ref_axis',(0.,0.,1.));
#4740=DIRECTION('center_axis',(-1.,-3.43024899888577E-15,1.22464679914735E-16));
#4741=DIRECTION('ref_axis',(-1.22464679914735E-16,0.,-1.));
#4742=DIRECTION('center_axis',(-3.43024899888577E-15,1.,0.));
#4743=DIRECTION('ref_axis',(0.,0.,1.));
#4744=DIRECTION('center_axis',(-1.,-3.43024899888577E-15,1.22464679914735E-16));
#4745=DIRECTION('ref_axis',(-1.22464679914735E-16,0.,-1.));
#5571=CARTESIAN_POINT('',(0.,0.,0.));
#5572=CARTESIAN_POINT('Origin',(-2.22044604925031E-13,65.9999999999997,
0.));
#5573=CARTESIAN_POINT('',(84.5218814663268,63.9999999999999,24.4959497344398));
#5574=CARTESIAN_POINT('',(84.5218814663268,63.9999999999999,-24.4959497344398));
#5575=CARTESIAN_POINT('Origin',(-2.19535935928688E-13,63.9999999999996,
0.));
#5576=CARTESIAN_POINT('',(89.1964124839111,65.9999999999999,12.));
#5577=CARTESIAN_POINT('Ctrl Pts',(84.5218814663268,64.,24.4959497344398));
#5578=CARTESIAN_POINT('Ctrl Pts',(84.9038127722375,64.,23.9157900880511));
#5579=CARTESIAN_POINT('Ctrl Pts',(85.2940373732189,64.0317096659725,23.2792569494813));
#5580=CARTESIAN_POINT('Ctrl Pts',(87.3160364923004,64.3594769795007,19.6445825482463));
#5581=CARTESIAN_POINT('Ctrl Pts',(88.643006529544,65.1313887892092,16.0828655187997));
#5582=CARTESIAN_POINT('Ctrl Pts',(89.1937556100172,65.9958068625112,12.0197115471009));
#5583=CARTESIAN_POINT('Ctrl Pts',(89.1950864974236,65.9979034312765,12.0098561031404));
#5584=CARTESIAN_POINT('Ctrl Pts',(89.196412483911,66.,12.));
#5585=CARTESIAN_POINT('',(-90.0000000000005,65.9999999999993,-1.10218211923262E-14));
#5586=CARTESIAN_POINT('Origin',(-2.2639643392646E-13,65.9999999999996,0.));
#5587=CARTESIAN_POINT('',(89.196412483911,65.9999999999999,-12.));
#5588=CARTESIAN_POINT('Origin',(-2.2639643392646E-13,65.9999999999996,0.));
#5589=CARTESIAN_POINT('Ctrl Pts',(84.5218814663268,64.,-24.4959497344398));
#5590=CARTESIAN_POINT('Ctrl Pts',(84.7701310773201,64.,-24.1188546801693));
#5591=CARTESIAN_POINT('Ctrl Pts',(85.0220290607656,64.0133758231304,-23.7177022308239));
#5592=CARTESIAN_POINT('Ctrl Pts',(86.1522258688305,64.1327263249616,-21.8101284980407));
#5593=CARTESIAN_POINT('Ctrl Pts',(86.9849682511504,64.379237185943,-20.1156541149184));
#5594=CARTESIAN_POINT('Ctrl Pts',(88.4016861752627,65.0999401070311,-16.1941739449509));
#5595=CARTESIAN_POINT('Ctrl Pts',(88.9080060701816,65.5473139367667,-14.1278301420605));
#5596=CARTESIAN_POINT('Ctrl Pts',(89.1937556100206,65.9958068625089,-12.0197115470756));
#5597=CARTESIAN_POINT('Ctrl Pts',(89.195086497424,65.9979034312771,-12.0098561031374));
#5598=CARTESIAN_POINT('Ctrl Pts',(89.196412483911,66.,-12.));
#5599=CARTESIAN_POINT('Origin',(-90.0010000000005,21.9999999999997,0.));
#5600=CARTESIAN_POINT('',(41.13395568512,21.9999999999999,38.));
#5601=CARTESIAN_POINT('',(41.1339720798708,21.9999999999999,-38.));
#5602=CARTESIAN_POINT('Ctrl Pts',(41.13395568512,21.9999999999997,38.));
#5603=CARTESIAN_POINT('Ctrl Pts',(41.13395568512,24.5049526391433,38.));
#5604=CARTESIAN_POINT('Ctrl Pts',(41.3698859733185,27.0457064732876,37.7490333835055));
#5605=CARTESIAN_POINT('Ctrl Pts',(42.2668103555191,32.0237155256726,36.7419897039594));
#5606=CARTESIAN_POINT('Ctrl Pts',(42.9248433632201,34.4616282231014,35.9865277696606));
#5607=CARTESIAN_POINT('Ctrl Pts',(44.4913270859975,39.0947019839386,34.0307796957095));
#5608=CARTESIAN_POINT('Ctrl Pts',(45.398690949306,41.2947913266836,32.8288186947832));
#5609=CARTESIAN_POINT('Ctrl Pts',(47.2681227122205,45.3564353734818,30.0748605376039));
#5610=CARTESIAN_POINT('Ctrl Pts',(48.2290184872111,47.2180132517743,28.5221020796692));
#5611=CARTESIAN_POINT('Ctrl Pts',(50.0250804079731,50.5021494267391,25.2379659817043));
#5612=CARTESIAN_POINT('Ctrl Pts',(50.9300602235279,52.0511318891308,23.387202355214));
#5613=CARTESIAN_POINT('Ctrl Pts',(52.6061045330048,54.8116067028424,19.3243428839503));
#5614=CARTESIAN_POINT('Ctrl Pts',(53.3762495117073,56.0232593397458,17.1119766759343));
#5615=CARTESIAN_POINT('Ctrl Pts',(54.6519856594464,57.9916316933046,12.4500772721613));
#5616=CARTESIAN_POINT('Ctrl Pts',(55.1581885566719,58.7499727721315,9.99553864743798));
#5617=CARTESIAN_POINT('Ctrl Pts',(55.8324050725756,59.7543646835585,5.00791763065262));
#5618=CARTESIAN_POINT('Ctrl Pts',(56.0000358879638,59.9999999999997,2.47469983355769));
#5619=CARTESIAN_POINT('Ctrl Pts',(56.0000366722163,59.9999999999997,-2.47469958668799));
#5620=CARTESIAN_POINT('Ctrl Pts',(55.8324066922941,59.7543647315935,-5.00791719772311));
#5621=CARTESIAN_POINT('Ctrl Pts',(55.1581918868508,58.7499729504375,-9.99553795640079));
#5622=CARTESIAN_POINT('Ctrl Pts',(54.6519898647332,57.9916319532894,-12.4500765088443));
#5623=CARTESIAN_POINT('Ctrl Pts',(53.3762554539761,56.0232597504026,-17.1119758509008));
#5624=CARTESIAN_POINT('Ctrl Pts',(52.6061113388684,54.8116071817857,-19.3243420707035));
#5625=CARTESIAN_POINT('Ctrl Pts',(50.9300687027128,52.0511324690522,-23.3872016100264));
#5626=CARTESIAN_POINT('Ctrl Pts',(50.0250896973938,50.5021500393159,-25.2379652925953));
#5627=CARTESIAN_POINT('Ctrl Pts',(48.2290292589987,47.2180138110437,-28.5221015978674));
#5628=CARTESIAN_POINT('Ctrl Pts',(47.2681342172102,45.3564358424301,-30.0748601848596));
#5629=CARTESIAN_POINT('Ctrl Pts',(45.3987038776794,41.2947915957089,-32.8288185471517));
#5630=CARTESIAN_POINT('Ctrl Pts',(44.4913407056712,39.0947021428606,-34.030779623489));
#5631=CARTESIAN_POINT('Ctrl Pts',(42.9248582173494,34.4616281959662,-35.9865277862501));
#5632=CARTESIAN_POINT('Ctrl Pts',(42.2668257527207,32.0237154223944,-36.7419897336045));
#5633=CARTESIAN_POINT('Ctrl Pts',(41.369902143272,27.0457063249303,-37.7490334047659));
#5634=CARTESIAN_POINT('Ctrl Pts',(41.1339720798708,24.504952523231,-38.));
#5635=CARTESIAN_POINT('Ctrl Pts',(41.1339720798708,21.9999999999997,-38.));
#5636=CARTESIAN_POINT('',(59.4642749892742,22.,-38.));
#5637=CARTESIAN_POINT('',(41.1339720798708,21.9999999999999,-38.));
#5638=CARTESIAN_POINT('',(89.1964124839111,58.0555127546396,-12.));
#5639=CARTESIAN_POINT('Ctrl Pts',(89.1964124839111,58.0555127546396,-12.));
#5640=CARTESIAN_POINT('Ctrl Pts',(89.1190199896171,57.8640542974771,-12.5752610703505));
#5641=CARTESIAN_POINT('Ctrl Pts',(89.0250779102713,57.6584422520644,-13.1470340093289));
#5642=CARTESIAN_POINT('Ctrl Pts',(88.5525797543681,56.7159929487085,-15.5825558333806));
#5643=CARTESIAN_POINT('Ctrl Pts',(88.0143914281752,55.8427290142663,-17.3935784710887));
#5644=CARTESIAN_POINT('Ctrl Pts',(86.6610431662391,53.8665957514274,-20.7939147542697));
#5645=CARTESIAN_POINT('Ctrl Pts',(85.8451876894935,52.76239978252,-22.3861978423013));
#5646=CARTESIAN_POINT('Ctrl Pts',(84.0425817165657,50.4264221335801,-25.2864710591156));
#5647=CARTESIAN_POINT('Ctrl Pts',(83.056053899723,49.1947849510484,-26.5947159612042));
#5648=CARTESIAN_POINT('Ctrl Pts',(80.5654234362146,46.1505453853588,-29.4436626273688));
#5649=CARTESIAN_POINT('Ctrl Pts',(78.8977661523696,44.1685496793139,-30.9617789456884));
#5650=CARTESIAN_POINT('Ctrl Pts',(75.3156320753682,39.9826685922426,-33.5663519067529));
#5651=CARTESIAN_POINT('Ctrl Pts',(73.4012521028471,37.7788157607244,-34.6529940162392));
#5652=CARTESIAN_POINT('Ctrl Pts',(69.4585378993709,33.2773576738104,-36.367872488476));
#5653=CARTESIAN_POINT('Ctrl Pts',(67.429009853746,30.978347996818,-36.9965695983663));
#5654=CARTESIAN_POINT('Ctrl Pts',(63.3934115878716,26.4218766001607,-37.8127478744626));
#5655=CARTESIAN_POINT('Ctrl Pts',(61.3873583010373,24.164358858964,-38.));
#5656=CARTESIAN_POINT('Ctrl Pts',(59.4642749892743,21.9999999999999,-38.));
#5657=CARTESIAN_POINT('',(89.1964124839111,58.0555127546396,12.));
#5658=CARTESIAN_POINT('Ctrl Pts',(89.1964124839111,58.0555127546396,-12.));
#5659=CARTESIAN_POINT('Ctrl Pts',(89.4006007095317,58.5606465276845,-10.4822619002651));
#5660=CARTESIAN_POINT('Ctrl Pts',(89.5691633283084,58.9690896845165,-8.93349037421489));
#5661=CARTESIAN_POINT('Ctrl Pts',(89.9001752372116,59.765576470203,-4.90814187236786));
#5662=CARTESIAN_POINT('Ctrl Pts',(90.0000000000001,59.9999999999997,-2.41748397242429));
#5663=CARTESIAN_POINT('Ctrl Pts',(90.0000000000001,59.9999999999997,2.41748397242427));
#5664=CARTESIAN_POINT('Ctrl Pts',(89.9001752372116,59.7655764702031,4.90814187236785));
#5665=CARTESIAN_POINT('Ctrl Pts',(89.5691633283084,58.9690896845165,8.93349037421488));
#5666=CARTESIAN_POINT('Ctrl Pts',(89.4006007095317,58.5606465276845,10.4822619002651));
#5667=CARTESIAN_POINT('Ctrl Pts',(89.1964124839111,58.0555127546396,12.));
#5668=CARTESIAN_POINT('',(59.4642749892742,22.,38.));
#5669=CARTESIAN_POINT('Ctrl Pts',(89.1964124839111,58.0555127546396,12.));
#5670=CARTESIAN_POINT('Ctrl Pts',(89.1190199896171,57.8640542974771,12.5752610703505));
#5671=CARTESIAN_POINT('Ctrl Pts',(89.0250779102713,57.6584422520644,13.1470340093289));
#5672=CARTESIAN_POINT('Ctrl Pts',(88.5525797543681,56.7159929487085,15.5825558333806));
#5673=CARTESIAN_POINT('Ctrl Pts',(88.0143914281752,55.8427290142662,17.3935784710887));
#5674=CARTESIAN_POINT('Ctrl Pts',(86.6610431662391,53.8665957514274,20.7939147542697));
#5675=CARTESIAN_POINT('Ctrl Pts',(85.8451876894935,52.76239978252,22.3861978423013));
#5676=CARTESIAN_POINT('Ctrl Pts',(84.0425817165657,50.4264221335801,25.2864710591156));
#5677=CARTESIAN_POINT('Ctrl Pts',(83.0560538997229,49.1947849510483,26.5947159612043));
#5678=CARTESIAN_POINT('Ctrl Pts',(80.5654234362146,46.1505453853588,29.4436626273688));
#5679=CARTESIAN_POINT('Ctrl Pts',(78.8977661523695,44.1685496793138,30.9617789456885));
#5680=CARTESIAN_POINT('Ctrl Pts',(75.3156320753681,39.9826685922425,33.5663519067529));
#5681=CARTESIAN_POINT('Ctrl Pts',(73.4012521028471,37.7788157607244,34.6529940162392));
#5682=CARTESIAN_POINT('Ctrl Pts',(69.4585378993709,33.2773576738104,36.367872488476));
#5683=CARTESIAN_POINT('Ctrl Pts',(67.429009853746,30.978347996818,36.9965695983663));
#5684=CARTESIAN_POINT('Ctrl Pts',(63.3934115878716,26.4218766001607,37.8127478744626));
#5685=CARTESIAN_POINT('Ctrl Pts',(61.3873583010373,24.164358858964,38.));
#5686=CARTESIAN_POINT('Ctrl Pts',(59.4642749892743,21.9999999999999,38.));
#5687=CARTESIAN_POINT('',(114.,21.9999999999997,38.));
#5688=CARTESIAN_POINT('',(-90.0010000000005,21.9999999999997,38.));
#5689=CARTESIAN_POINT('Origin',(114.,21.9999999999997,0.));
#5690=CARTESIAN_POINT('',(59.4642749892742,22.,38.));
#5691=CARTESIAN_POINT('',(52.1152568831818,-10.0000000000004,20.493901531919));
#5692=CARTESIAN_POINT('Ctrl Pts',(41.1339276024063,21.9999999999997,38.));
#5693=CARTESIAN_POINT('Ctrl Pts',(41.1339276024063,19.4950474188123,38.));
#5694=CARTESIAN_POINT('Ctrl Pts',(41.3698577782062,16.9542936008905,37.7490333941357));
#5695=CARTESIAN_POINT('Ctrl Pts',(42.2667817740307,11.9762845259659,36.741989718782));
#5696=CARTESIAN_POINT('Ctrl Pts',(42.9248145101955,9.53837179046566,35.9865277779553));
#5697=CARTESIAN_POINT('Ctrl Pts',(44.491297615745,4.90529793659982,34.0307796595992));
#5698=CARTESIAN_POINT('Ctrl Pts',(45.3986611334033,2.70520853880316,32.8288186209674));
#5699=CARTESIAN_POINT('Ctrl Pts',(47.2680921846259,-1.3564356079566,30.0748603612317));
#5700=CARTESIAN_POINT('Ctrl Pts',(48.2289875930154,-3.21801353140966,28.5221018387682));
#5701=CARTESIAN_POINT('Ctrl Pts',(50.0250487725939,-6.50214973302819,25.2379656371497));
#5702=CARTESIAN_POINT('Ctrl Pts',(50.9300281830307,-8.05113217909215,23.3872019826201));
#5703=CARTESIAN_POINT('Ctrl Pts',(51.8851439691307,-9.62422563773273,21.0719271623962));
#5704=CARTESIAN_POINT('Ctrl Pts',(52.0009460104357,-9.81383310944727,20.7845899832333));
#5705=CARTESIAN_POINT('Ctrl Pts',(52.1152568831818,-10.0000000000004,20.493901531919));
#5706=CARTESIAN_POINT('',(52.1152568831817,-10.0000000000002,-20.4939015319188));
#5707=CARTESIAN_POINT('Ctrl Pts',(52.1152568831816,-10.0000000000005,20.493901531919));
#5708=CARTESIAN_POINT('Ctrl Pts',(52.9920598772145,-11.427962914687,18.2642229517423));
#5709=CARTESIAN_POINT('Ctrl Pts',(53.4487275116836,-12.800109304042,15.628623783461));
#5710=CARTESIAN_POINT('Ctrl Pts',(53.6428401425395,-14.8055170663448,9.84683279520228));
#5711=CARTESIAN_POINT('Ctrl Pts',(53.4915500984615,-15.4263415985926,7.14093283352039));
#5712=CARTESIAN_POINT('Ctrl Pts',(53.3537086148268,-15.8453555314119,3.53009503335275));
#5713=CARTESIAN_POINT('Ctrl Pts',(53.3258483126282,-15.9159138020226,2.67163594799237));
#5714=CARTESIAN_POINT('Ctrl Pts',(53.2987508848524,-15.9829447710969,1.26141826952118));
#5715=CARTESIAN_POINT('Ctrl Pts',(53.2926607217507,-15.9972472233255,0.715583753770389));
#5716=CARTESIAN_POINT('Ctrl Pts',(53.2906987538236,-16.0019108788503,-0.356739054022367));
#5717=CARTESIAN_POINT('Ctrl Pts',(53.294321434229,-15.99345855971,-0.881048064909989));
#5718=CARTESIAN_POINT('Ctrl Pts',(53.3135705802987,-15.9465857713104,-2.14429489073831));
#5719=CARTESIAN_POINT('Ctrl Pts',(53.3333698832412,-15.8978903517419,-2.88150257955492));
#5720=CARTESIAN_POINT('Ctrl Pts',(53.3892695140974,-15.7411204686839,-4.51882129056692));
#5721=CARTESIAN_POINT('Ctrl Pts',(53.4277924573997,-15.6228736964551,-5.41747303556089));
#5722=CARTESIAN_POINT('Ctrl Pts',(53.5329994424471,-15.1901728977435,-7.98473738653545));
#5723=CARTESIAN_POINT('Ctrl Pts',(53.5944639440763,-14.7956338714779,-9.64539296566124));
#5724=CARTESIAN_POINT('Ctrl Pts',(53.5480496875213,-13.1924305377066,-14.7997725951247));
#5725=CARTESIAN_POINT('Ctrl Pts',(53.1488326938255,-11.7260326931231,-17.7622050761178));
#5726=CARTESIAN_POINT('Ctrl Pts',(52.1679065869839,-10.0863024534087,-20.358676489776));
#5727=CARTESIAN_POINT('Ctrl Pts',(52.141763209695,-10.0431682504778,-20.4264968938551));
#5728=CARTESIAN_POINT('Ctrl Pts',(52.1152568831816,-10.0000000000005,-20.493901531919));
#5729=CARTESIAN_POINT('Ctrl Pts',(52.1152568831818,-10.0000000000004,-20.493901531919));
#5730=CARTESIAN_POINT('Ctrl Pts',(52.0009460104357,-9.81383310944727,-20.7845899832333));
#5731=CARTESIAN_POINT('Ctrl Pts',(51.8851439691307,-9.62422563773273,-21.0719271623962));
#5732=CARTESIAN_POINT('Ctrl Pts',(50.9300281830307,-8.05113217909215,-23.3872019826201));
#5733=CARTESIAN_POINT('Ctrl Pts',(50.0250487725939,-6.50214973302819,-25.2379656371497));
#5734=CARTESIAN_POINT('Ctrl Pts',(48.2289875930154,-3.21801353140967,-28.5221018387682));
#5735=CARTESIAN_POINT('Ctrl Pts',(47.2680921846259,-1.3564356079566,-30.0748603612317));
#5736=CARTESIAN_POINT('Ctrl Pts',(45.3986611334033,2.70520853880316,-32.8288186209674));
#5737=CARTESIAN_POINT('Ctrl Pts',(44.491297615745,4.90529793659981,-34.0307796595992));
#5738=CARTESIAN_POINT('Ctrl Pts',(42.9248145101955,9.53837179046566,-35.9865277779553));
#5739=CARTESIAN_POINT('Ctrl Pts',(42.2667817740307,11.9762845259659,-36.741989718782));
#5740=CARTESIAN_POINT('Ctrl Pts',(41.3698577782062,16.9542936008905,-37.7490333941357));
#5741=CARTESIAN_POINT('Ctrl Pts',(41.1339276024063,19.4950474188123,-38.));
#5742=CARTESIAN_POINT('Ctrl Pts',(41.1339276024063,24.5049525811872,-38.));
#5743=CARTESIAN_POINT('Ctrl Pts',(41.3698577782062,27.045706399109,-37.7490333941357));
#5744=CARTESIAN_POINT('Ctrl Pts',(42.2667817740307,32.0237154740336,-36.741989718782));
#5745=CARTESIAN_POINT('Ctrl Pts',(42.9248145101955,34.4616282095338,-35.9865277779553));
#5746=CARTESIAN_POINT('Ctrl Pts',(44.4912976157449,39.0947020633997,-34.0307796595992));
#5747=CARTESIAN_POINT('Ctrl Pts',(45.3986611334032,41.2947914611964,-32.8288186209674));
#5748=CARTESIAN_POINT('Ctrl Pts',(47.2680921846258,45.3564356079561,-30.0748603612317));
#5749=CARTESIAN_POINT('Ctrl Pts',(48.2289875930153,47.2180135314092,-28.5221018387682));
#5750=CARTESIAN_POINT('Ctrl Pts',(50.0250487725937,50.5021497330277,-25.2379656371497));
#5751=CARTESIAN_POINT('Ctrl Pts',(50.9300281830306,52.0511321790916,-23.38720198262));
#5752=CARTESIAN_POINT('Ctrl Pts',(52.6060716558467,54.8116069423141,-19.3243424773267));
#5753=CARTESIAN_POINT('Ctrl Pts',(53.3762162027518,56.0232595450743,-17.1119762634174));
#5754=CARTESIAN_POINT('Ctrl Pts',(54.6519514819998,57.991631823297,-12.4500768905027));
#5755=CARTESIAN_POINT('Ctrl Pts',(55.1581539416713,58.7499728612845,-9.99553830191928));
#5756=CARTESIAN_POINT('Ctrl Pts',(55.8323696023447,59.754364707576,-5.0079174141878));
#5757=CARTESIAN_POINT('Ctrl Pts',(55.9999999999999,59.9999999999997,-2.47469971012283));
#5758=CARTESIAN_POINT('Ctrl Pts',(55.9999999999999,59.9999999999997,2.4746997101228));
#5759=CARTESIAN_POINT('Ctrl Pts',(55.8323696023447,59.754364707576,5.00791741418778));
#5760=CARTESIAN_POINT('Ctrl Pts',(55.1581539416713,58.7499728612845,9.99553830191926));
#5761=CARTESIAN_POINT('Ctrl Pts',(54.6519514819998,57.991631823297,12.4500768905027));
#5762=CARTESIAN_POINT('Ctrl Pts',(53.3762162027518,56.0232595450743,17.1119762634174));
#5763=CARTESIAN_POINT('Ctrl Pts',(52.6060716558467,54.8116069423141,19.3243424773267));
#5764=CARTESIAN_POINT('Ctrl Pts',(50.9300281830306,52.0511321790916,23.38720198262));
#5765=CARTESIAN_POINT('Ctrl Pts',(50.0250487725937,50.5021497330277,25.2379656371497));
#5766=CARTESIAN_POINT('Ctrl Pts',(48.2289875930153,47.2180135314091,28.5221018387682));
#5767=CARTESIAN_POINT('Ctrl Pts',(47.2680921846258,45.3564356079561,30.0748603612317));
#5768=CARTESIAN_POINT('Ctrl Pts',(45.3986611334032,41.2947914611964,32.8288186209674));
#5769=CARTESIAN_POINT('Ctrl Pts',(44.491297615745,39.0947020633997,34.0307796595992));
#5770=CARTESIAN_POINT('Ctrl Pts',(42.9248145101955,34.4616282095338,35.9865277779553));
#5771=CARTESIAN_POINT('Ctrl Pts',(42.2667817740307,32.0237154740336,36.741989718782));
#5772=CARTESIAN_POINT('Ctrl Pts',(41.3698577782062,27.045706399109,37.7490333941357));
#5773=CARTESIAN_POINT('Ctrl Pts',(41.1339276024063,24.5049525811872,38.));
#5774=CARTESIAN_POINT('Ctrl Pts',(41.1339276024063,21.9999999999997,38.));
#5775=CARTESIAN_POINT('Origin',(-2.15105711021124E-13,61.9999999999998,
0.));
#5776=CARTESIAN_POINT('',(-56.0000000000003,61.9999999999996,-6.85802207522519E-15));
#5777=CARTESIAN_POINT('',(-2.21963733096349E-13,61.9999999999997,56.0000000000002));
#5778=CARTESIAN_POINT('Origin',(-2.12675437930917E-13,61.9999999999997,
0.));
#5779=CARTESIAN_POINT('Origin',(-2.12675437930917E-13,61.9999999999997,
0.));
#5780=CARTESIAN_POINT('',(-2.2906916045395E-13,63.9999999999997,58.0000000000002));
#5781=CARTESIAN_POINT('Origin',(-2.22208662456179E-13,61.9999999999998,
58.0000000000002));
#5782=CARTESIAN_POINT('',(43.8178046004133,63.9999999999999,-38.));
#5783=CARTESIAN_POINT('Origin',(-2.19535935928689E-13,63.9999999999997,
0.));
#5784=CARTESIAN_POINT('',(41.1339720798706,62.0114315300489,-38.));
#5785=CARTESIAN_POINT('Ctrl Pts',(43.8178046004133,63.9999999999999,-38.));
#5786=CARTESIAN_POINT('Ctrl Pts',(43.4594642227257,63.9999999999999,-38.));
#5787=CARTESIAN_POINT('Ctrl Pts',(43.0349690410079,63.9313624698626,-38.));
#5788=CARTESIAN_POINT('Ctrl Pts',(42.398381143829,63.7105066153047,-38.));
#5789=CARTESIAN_POINT('Ctrl Pts',(42.0643495443749,63.5323654074303,-38.));
#5790=CARTESIAN_POINT('Ctrl Pts',(41.6188649978616,63.1625011801094,-38.));
#5791=CARTESIAN_POINT('Ctrl Pts',(41.4150926413892,62.9206514303181,-38.));
#5792=CARTESIAN_POINT('Ctrl Pts',(41.2006682164102,62.4874233680621,-38.));
#5793=CARTESIAN_POINT('Ctrl Pts',(41.1356921995111,62.232481043002,-38.));
#5794=CARTESIAN_POINT('Ctrl Pts',(41.1339720798706,62.0114315300489,-38.));
#5795=CARTESIAN_POINT('',(41.1339556851194,62.0090835271345,38.));
#5796=CARTESIAN_POINT('Ctrl Pts',(41.1339720798707,62.0114315300484,-38.));
#5797=CARTESIAN_POINT('Ctrl Pts',(41.5378675708182,62.011465189054,-37.5627943401587));
#5798=CARTESIAN_POINT('Ctrl Pts',(41.9345050198156,62.0114977099643,-37.1194669610288));
#5799=CARTESIAN_POINT('Ctrl Pts',(42.3240191945377,62.0115291274321,-36.6698939326639));
#5800=CARTESIAN_POINT('Ctrl Pts',(42.508108342725,62.0115439757104,-36.4574202379678));
#5801=CARTESIAN_POINT('Ctrl Pts',(42.6906058723339,62.0115585775212,-36.243550982485));
#5802=CARTESIAN_POINT('Ctrl Pts',(42.8715229676726,62.0115729365226,-36.028270407902));
#5803=CARTESIAN_POINT('Ctrl Pts',(43.1691570145251,62.0115965590979,-35.6741036084522));
#5804=CARTESIAN_POINT('Ctrl Pts',(43.4625105062847,62.0116195245126,-35.316113143293));
#5805=CARTESIAN_POINT('Ctrl Pts',(43.7511863459427,62.0116418174384,-34.95479206422));
#5806=CARTESIAN_POINT('Ctrl Pts',(44.0092631669743,62.011661747362,-34.6317702430334));
#5807=CARTESIAN_POINT('Ctrl Pts',(44.2636018952112,62.0116811398056,-34.3060870015161));
#5808=CARTESIAN_POINT('Ctrl Pts',(44.513946804719,62.011699983817,-33.9781160868287));
#5809=CARTESIAN_POINT('Ctrl Pts',(44.9124183662909,62.0117299776468,-33.4560879665742));
#5810=CARTESIAN_POINT('Ctrl Pts',(45.3007823806485,62.0117585820355,-32.9282686995972));
#5811=CARTESIAN_POINT('Ctrl Pts',(45.6791840228587,62.0117858374024,-32.3946914848435));
#5812=CARTESIAN_POINT('Ctrl Pts',(46.0592450736997,62.0118132122926,-31.8587743684177));
#5813=CARTESIAN_POINT('Ctrl Pts',(46.4292564142946,62.0118392263032,-31.3170484260819));
#5814=CARTESIAN_POINT('Ctrl Pts',(46.7893273274975,62.0118639203879,-30.7695107101662));
#5815=CARTESIAN_POINT('Ctrl Pts',(47.0250930021408,62.0118800894739,-30.4109963335472));
#5816=CARTESIAN_POINT('Ctrl Pts',(47.2565961247388,62.0118956926664,-30.0499895290226));
#5817=CARTESIAN_POINT('Ctrl Pts',(47.4838579530542,62.0119107414621,-29.686481875962));
#5818=CARTESIAN_POINT('Ctrl Pts',(47.8495677822757,62.0119349579904,-29.1015252085492));
#5819=CARTESIAN_POINT('Ctrl Pts',(48.204293167232,62.0119577388937,-28.5100992575856));
#5820=CARTESIAN_POINT('Ctrl Pts',(48.5480436433421,62.01197910361,-27.9122101670856));
#5821=CARTESIAN_POINT('Ctrl Pts',(48.6366313782987,62.0119846094987,-27.7581285178557));
#5822=CARTESIAN_POINT('Ctrl Pts',(48.7244899943061,62.0119900213324,-27.6036174841194));
#5823=CARTESIAN_POINT('Ctrl Pts',(48.8116191692164,62.0119953394441,-27.4486768895265));
#5824=CARTESIAN_POINT('Ctrl Pts',(49.2076260972417,62.0120195105561,-26.7444633014341));
#5825=CARTESIAN_POINT('Ctrl Pts',(49.5885686299212,62.0120417456002,-26.031376792441));
#5826=CARTESIAN_POINT('Ctrl Pts',(49.9542510971775,62.0120620654678,-25.3096201309785));
#5827=CARTESIAN_POINT('Ctrl Pts',(49.9812271085838,62.0120635644431,-25.2563769003739));
#5828=CARTESIAN_POINT('Ctrl Pts',(50.0081200547548,62.0120650529963,-25.2030864800111));
#5829=CARTESIAN_POINT('Ctrl Pts',(50.0349298464748,62.0120665311357,-25.1497489476434));
#5830=CARTESIAN_POINT('Ctrl Pts',(50.2703252167996,62.0120795094975,-24.681434672209));
#5831=CARTESIAN_POINT('Ctrl Pts',(50.4993133690921,62.0120916850446,-24.2094914308971));
#5832=CARTESIAN_POINT('Ctrl Pts',(50.7219802963322,62.0121030623635,-23.7336220668136));
#5833=CARTESIAN_POINT('Ctrl Pts',(50.868451137173,62.0121105463912,-23.4205940533962));
#5834=CARTESIAN_POINT('Ctrl Pts',(51.012185793409,62.0121176850223,-23.1058667532725));
#5835=CARTESIAN_POINT('Ctrl Pts',(51.1531972464791,62.0121244795624,-22.789351188351));
#5836=CARTESIAN_POINT('Ctrl Pts',(51.3210673250925,62.0121325682669,-22.4125485130439));
#5837=CARTESIAN_POINT('Ctrl Pts',(51.4850732756592,62.012140169318,-22.0332086150571));
#5838=CARTESIAN_POINT('Ctrl Pts',(51.6449228820795,62.0121472726493,-21.6519299860615));
#5839=CARTESIAN_POINT('Ctrl Pts',(51.8047054217536,62.0121543730003,-21.2708113269125));
#5840=CARTESIAN_POINT('Ctrl Pts',(51.9603350272497,62.0121609760492,-20.8877557340995));
#5841=CARTESIAN_POINT('Ctrl Pts',(52.1115677050986,62.0121670717421,-20.5033815847748));
#5842=CARTESIAN_POINT('Ctrl Pts',(52.1293310215895,62.0121677877231,-20.458234201534));
#5843=CARTESIAN_POINT('Ctrl Pts',(52.1470337325548,62.0121684967045,-20.4130686489935));
#5844=CARTESIAN_POINT('Ctrl Pts',(52.1646754866477,62.0121691986701,-20.3678859461551));
#5845=CARTESIAN_POINT('Ctrl Pts',(52.4827757330314,62.0121818558829,-19.5531920767413));
#5846=CARTESIAN_POINT('Ctrl Pts',(52.7810569708954,62.0121922321038,-18.7329183662393));
#5847=CARTESIAN_POINT('Ctrl Pts',(53.0594801179139,62.0122003722445,-17.9079797138351));
#5848=CARTESIAN_POINT('Ctrl Pts',(53.2654855976632,62.0122063951403,-17.2976070322818));
#5849=CARTESIAN_POINT('Ctrl Pts',(53.4606249872914,62.0122111938872,-16.6846825185638));
#5850=CARTESIAN_POINT('Ctrl Pts',(53.645006030693,62.0122147829815,-16.0691476324579));
#5851=CARTESIAN_POINT('Ctrl Pts',(53.7098220009675,62.0122160446656,-15.8527669777835));
#5852=CARTESIAN_POINT('Ctrl Pts',(53.7733080750946,62.0122171568666,-15.6360635542535));
#5853=CARTESIAN_POINT('Ctrl Pts',(53.8354675204326,62.0122181202142,-15.4190342371275));
#5854=CARTESIAN_POINT('Ctrl Pts',(54.0249493601744,62.0122210568053,-14.7574595711486));
#5855=CARTESIAN_POINT('Ctrl Pts',(54.2021067755319,62.0122226102135,-14.0928599079471));
#5856=CARTESIAN_POINT('Ctrl Pts',(54.3669672963198,62.0122227785237,-13.4252392951594));
#5857=CARTESIAN_POINT('Ctrl Pts',(54.5317686288195,62.0122229467735,-12.757858371783));
#5858=CARTESIAN_POINT('Ctrl Pts',(54.6842819835983,62.0122217309197,-12.0874582951485));
#5859=CARTESIAN_POINT('Ctrl Pts',(54.8244843840114,62.0122191290495,-11.4140305179011));
#5860=CARTESIAN_POINT('Ctrl Pts',(54.8978161216433,62.0122177681622,-11.0617995366224));
#5861=CARTESIAN_POINT('Ctrl Pts',(54.9677790714846,62.0122160280985,-10.7087400841896));
#5862=CARTESIAN_POINT('Ctrl Pts',(55.0343643255293,62.0122139085844,-10.3548500883884));
#5863=CARTESIAN_POINT('Ctrl Pts',(55.1738277395596,62.0122094692432,-9.61362430628843));
#5864=CARTESIAN_POINT('Ctrl Pts',(55.2984759194646,62.012203365266,-8.86875624929427));
#5865=CARTESIAN_POINT('Ctrl Pts',(55.4081555458839,62.0121955718983,-8.12037336202324));
#5866=CARTESIAN_POINT('Ctrl Pts',(55.4247934124446,62.0121943896823,-8.00684731328274));
#5867=CARTESIAN_POINT('Ctrl Pts',(55.4410867338072,62.012193168591,-7.89324038814436));
#5868=CARTESIAN_POINT('Ctrl Pts',(55.457034869806,62.012191908538,-7.77955303875739));
#5869=CARTESIAN_POINT('Ctrl Pts',(55.5175753408372,62.0121871252705,-7.34798625987619));
#5870=CARTESIAN_POINT('Ctrl Pts',(55.5731452267925,62.0121817805551,-6.91526060581588));
#5871=CARTESIAN_POINT('Ctrl Pts',(55.6237433222154,62.0121758616839,-6.48099760138376));
#5872=CARTESIAN_POINT('Ctrl Pts',(55.6634045101909,62.0121712221918,-6.14060165355911));
#5873=CARTESIAN_POINT('Ctrl Pts',(55.7000044146649,62.0121662299287,-5.79926035246736));
#5874=CARTESIAN_POINT('Ctrl Pts',(55.7334497888444,62.0121608936061,-5.45772072568573));
#5875=CARTESIAN_POINT('Ctrl Pts',(55.7426726331568,62.0121594220701,-5.36353828994967));
#5876=CARTESIAN_POINT('Ctrl Pts',(55.7516559017131,62.0121579243709,-5.26934080753018));
#5877=CARTESIAN_POINT('Ctrl Pts',(55.7603983329535,62.0121564006911,-5.1751440150118));
#5878=CARTESIAN_POINT('Ctrl Pts',(55.8175970056945,62.0121464317868,-4.55884731671826));
#5879=CARTESIAN_POINT('Ctrl Pts',(55.8644832568223,62.0121353507522,-3.94257835777548));
#5880=CARTESIAN_POINT('Ctrl Pts',(55.9011202625538,62.0121231749186,-3.32699092712286));
#5881=CARTESIAN_POINT('Ctrl Pts',(55.9162959151216,62.0121181314874,-3.07200445139562));
#5882=CARTESIAN_POINT('Ctrl Pts',(55.9297136672316,62.0121129002156,-2.81713486821982));
#5883=CARTESIAN_POINT('Ctrl Pts',(55.9413806163243,62.0121074823351,-2.56242840483791));
#5884=CARTESIAN_POINT('Ctrl Pts',(55.9687757179352,62.0120947606384,-1.9643535019748));
#5885=CARTESIAN_POINT('Ctrl Pts',(55.9865226639761,62.0120810100653,-1.36717903886914));
#5886=CARTESIAN_POINT('Ctrl Pts',(55.9947322782494,62.012066226294,-0.77073585089363));
#5887=CARTESIAN_POINT('Ctrl Pts',(55.998459676216,62.0120595140421,-0.499933709403522));
#5888=CARTESIAN_POINT('Ctrl Pts',(56.000220327323,62.012052588805,-0.229282197751845));
#5889=CARTESIAN_POINT('Ctrl Pts',(56.0000210920964,62.012045450178,0.0412349762717366));
#5890=CARTESIAN_POINT('Ctrl Pts',(55.9994875740913,62.0120263341508,0.765633896347442));
#5891=CARTESIAN_POINT('Ctrl Pts',(55.9849031765495,62.0120056879541,1.48906785379857));
#5892=CARTESIAN_POINT('Ctrl Pts',(55.9563530719782,62.0119834973098,2.2114637323107));
#5893=CARTESIAN_POINT('Ctrl Pts',(55.9507591585882,62.0119791494258,2.35300506949458));
#5894=CARTESIAN_POINT('Ctrl Pts',(55.9446289445313,62.0119747422508,2.49450657020774));
#5895=CARTESIAN_POINT('Ctrl Pts',(55.9379628370825,62.0119702756773,2.63596770169497));
#5896=CARTESIAN_POINT('Ctrl Pts',(55.9058777584782,62.0119487773196,3.31684354387251));
#5897=CARTESIAN_POINT('Ctrl Pts',(55.8613820941595,62.0119259029036,3.99678377855943));
#5898=CARTESIAN_POINT('Ctrl Pts',(55.8044873472033,62.0119016284166,4.67580561158339));
#5899=CARTESIAN_POINT('Ctrl Pts',(55.789231442081,62.0118951193926,4.85788028832961));
#5900=CARTESIAN_POINT('Ctrl Pts',(55.773083747807,62.0118885097029,5.03988891584848));
#5901=CARTESIAN_POINT('Ctrl Pts',(55.7560438508535,62.0118817988845,5.22183177609851));
#5902=CARTESIAN_POINT('Ctrl Pts',(55.6920225510572,62.0118565853918,5.90541680209062));
#5903=CARTESIAN_POINT('Ctrl Pts',(55.615410854639,62.0118299443551,6.58807330611238));
#5904=CARTESIAN_POINT('Ctrl Pts',(55.5261553576502,62.0118018392235,7.26979856450947));
#5905=CARTESIAN_POINT('Ctrl Pts',(55.5030591332503,62.011794566591,7.44620539745826));
#5906=CARTESIAN_POINT('Ctrl Pts',(55.4791160204489,62.0117871959234,7.62254982231334));
#5907=CARTESIAN_POINT('Ctrl Pts',(55.4543245380382,62.0117797265876,7.79883166888876));
#5908=CARTESIAN_POINT('Ctrl Pts',(55.3585683509376,62.011750876553,8.47971380427104));
#5909=CARTESIAN_POINT('Ctrl Pts',(55.2501595693073,62.0117205545226,9.15966304948901));
#5910=CARTESIAN_POINT('Ctrl Pts',(55.1289824351151,62.0116887132261,9.83865444210619));
#5911=CARTESIAN_POINT('Ctrl Pts',(55.0975453254334,62.0116804526055,10.0148058837531));
#5912=CARTESIAN_POINT('Ctrl Pts',(55.0652485912683,62.0116720897314,10.1908927684566));
#5913=CARTESIAN_POINT('Ctrl Pts',(55.032089672709,62.0116636237787,10.3669144595589));
#5914=CARTESIAN_POINT('Ctrl Pts',(54.9135687328307,62.0116333636639,10.9960741901775));
#5915=CARTESIAN_POINT('Ctrl Pts',(54.7840366361783,62.0116017866311,11.6244014107884));
#5916=CARTESIAN_POINT('Ctrl Pts',(54.6433306503092,62.0115688367575,12.25194527151));
#5917=CARTESIAN_POINT('Ctrl Pts',(54.5929324045582,62.0115570347306,12.4767197153037));
#5918=CARTESIAN_POINT('Ctrl Pts',(54.5411001729428,62.0115450565767,12.7013934683708));
#5919=CARTESIAN_POINT('Ctrl Pts',(54.4878249957722,62.011532899726,12.9259681060992));
#5920=CARTESIAN_POINT('Ctrl Pts',(54.4137006342804,62.0115159853046,13.2384297911268));
#5921=CARTESIAN_POINT('Ctrl Pts',(54.3367784741253,62.0114987249528,13.5506990328332));
#5922=CARTESIAN_POINT('Ctrl Pts',(54.2572438873394,62.0114811570873,13.8620047849093));
#5923=CARTESIAN_POINT('Ctrl Pts',(54.2283995452362,62.0114747858526,13.9749042161435));
#5924=CARTESIAN_POINT('Ctrl Pts',(54.1992120853552,62.0114683741721,14.0876770418473));
#5925=CARTESIAN_POINT('Ctrl Pts',(54.1696919905561,62.0114619238783,14.2002869055221));
#5926=CARTESIAN_POINT('Ctrl Pts',(54.0587740072792,62.0114376877235,14.6234040757373));
#5927=CARTESIAN_POINT('Ctrl Pts',(53.9431637590319,62.0114129064316,15.0442218079722));
#5928=CARTESIAN_POINT('Ctrl Pts',(53.8228416772755,62.0113875607373,15.4630315513008));
#5929=CARTESIAN_POINT('Ctrl Pts',(53.6191496499546,62.0113446532697,16.1720303022786));
#5930=CARTESIAN_POINT('Ctrl Pts',(53.4019500394013,62.011300128295,16.8752731946603));
#5931=CARTESIAN_POINT('Ctrl Pts',(53.1714548723221,62.0112539514119,17.5727042036621));
#5932=CARTESIAN_POINT('Ctrl Pts',(53.1296403304496,62.0112455743807,17.6992264145119));
#5933=CARTESIAN_POINT('Ctrl Pts',(53.0873880903754,62.0112371429847,17.8255573514516));
#5934=CARTESIAN_POINT('Ctrl Pts',(53.044699235177,62.0112286570187,17.9516966717651));
#5935=CARTESIAN_POINT('Ctrl Pts',(52.8304155607197,62.0111860603276,18.5848735729654));
#5936=CARTESIAN_POINT('Ctrl Pts',(52.6051347514235,62.0111420886329,19.2132228618125));
#5937=CARTESIAN_POINT('Ctrl Pts',(52.3689251517624,62.0110966991285,19.836812402838));
#5938=CARTESIAN_POINT('Ctrl Pts',(52.298685369297,62.0110832020101,20.0222442979523));
#5939=CARTESIAN_POINT('Ctrl Pts',(52.227478875668,62.0110695795231,20.2072552362763));
#5940=CARTESIAN_POINT('Ctrl Pts',(52.1553066088181,62.0110558305417,20.3918467787042));
#5941=CARTESIAN_POINT('Ctrl Pts',(51.8999966385941,62.0110071934105,21.0448408338706));
#5942=CARTESIAN_POINT('Ctrl Pts',(51.6326051540701,62.0109569733346,21.6925867841522));
#5943=CARTESIAN_POINT('Ctrl Pts',(51.3531674886488,62.0109051010724,22.3350737339108));
#5944=CARTESIAN_POINT('Ctrl Pts',(51.0738152139627,62.0108532446614,22.9773643521084));
#5945=CARTESIAN_POINT('Ctrl Pts',(50.7824239594258,62.0107997370736,23.6143995446689));
#5946=CARTESIAN_POINT('Ctrl Pts',(50.4789812557923,62.0107445091308,24.2461478145941));
#5947=CARTESIAN_POINT('Ctrl Pts',(50.3372425961395,62.0107187120545,24.5412386239791));
#5948=CARTESIAN_POINT('Ctrl Pts',(50.1928738366941,62.0106925396239,24.8351755838836));
#5949=CARTESIAN_POINT('Ctrl Pts',(50.0458702895881,62.0106659847888,25.127953604534));
#5950=CARTESIAN_POINT('Ctrl Pts',(49.7551858170679,62.0106134753197,25.706892182369));
#5951=CARTESIAN_POINT('Ctrl Pts',(49.4542054026347,62.0105594706101,26.2812943293165));
#5952=CARTESIAN_POINT('Ctrl Pts',(49.1428195444775,62.0105038711921,26.8511894802682));
#5953=CARTESIAN_POINT('Ctrl Pts',(48.8330311455835,62.010448557008,27.4181609779323));
#5954=CARTESIAN_POINT('Ctrl Pts',(48.5129435967346,62.0103916644357,27.9806718822024));
#5955=CARTESIAN_POINT('Ctrl Pts',(48.1824079257721,62.0103330955301,28.5387202958513));
#5956=CARTESIAN_POINT('Ctrl Pts',(47.9576449716585,62.010293268905,28.9181910187081));
#5957=CARTESIAN_POINT('Ctrl Pts',(47.7280500113292,62.0102526671523,29.2955976696472));
#5958=CARTESIAN_POINT('Ctrl Pts',(47.49356595267,62.0102112594757,29.670930431553));
#5959=CARTESIAN_POINT('Ctrl Pts',(47.2620846493753,62.0101703820573,30.0414567581269));
#5960=CARTESIAN_POINT('Ctrl Pts',(47.0258323928037,62.0101287192237,30.4099606921261));
#5961=CARTESIAN_POINT('Ctrl Pts',(46.7851812262161,62.0100863113628,30.7757967597325));
#5962=CARTESIAN_POINT('Ctrl Pts',(46.5445300596285,62.010043903502,31.141632827339));
#5963=CARTESIAN_POINT('Ctrl Pts',(46.2994801027285,62.0100007506138,31.5048008283505));
#5964=CARTESIAN_POINT('Ctrl Pts',(46.0504549827791,62.0099568930863,31.8646884781416));
#5965=CARTESIAN_POINT('Ctrl Pts',(45.7176003038583,62.0098982717583,32.3457254439829));
#5966=CARTESIAN_POINT('Ctrl Pts',(45.3776535651338,62.0098383915342,32.8209111895306));
#5967=CARTESIAN_POINT('Ctrl Pts',(45.0305386446111,62.009777170325,33.2904380565692));
#5968=CARTESIAN_POINT('Ctrl Pts',(44.8582657349873,62.0097467862786,33.5234639357492));
#5969=CARTESIAN_POINT('Ctrl Pts',(44.6842265206803,62.0097160719302,33.7550955348643));
#5970=CARTESIAN_POINT('Ctrl Pts',(44.5084077393491,62.0096850172446,33.9853537117308));
#5971=CARTESIAN_POINT('Ctrl Pts',(44.0783183399654,62.0096090510086,34.5486132238367));
#5972=CARTESIAN_POINT('Ctrl Pts',(43.6375851668711,62.0095310482173,35.1036522194153));
#5973=CARTESIAN_POINT('Ctrl Pts',(43.1862189041955,62.0094508349908,35.6504277348031));
#5974=CARTESIAN_POINT('Ctrl Pts',(42.7359482888616,62.0093708164741,36.1958760062442));
#5975=CARTESIAN_POINT('Ctrl Pts',(42.2750958715132,62.0092885982405,36.7331011603559));
#5976=CARTESIAN_POINT('Ctrl Pts',(41.8036345689526,62.009204007673,37.2620250230665));
#5977=CARTESIAN_POINT('Ctrl Pts',(41.582739475743,62.009164374216,37.5098432115788));
#5978=CARTESIAN_POINT('Ctrl Pts',(41.3595149744804,62.0091242199772,37.7558385404457));
#5979=CARTESIAN_POINT('Ctrl Pts',(41.1339556851197,62.0090835272022,38.0000000000002));
#5980=CARTESIAN_POINT('',(43.8178046004133,63.9999999999999,38.));
#5981=CARTESIAN_POINT('Ctrl Pts',(41.1339556851194,62.0090835271345,38.));
#5982=CARTESIAN_POINT('Ctrl Pts',(41.1353258249379,62.2306725157175,38.));
#5983=CARTESIAN_POINT('Ctrl Pts',(41.2003227396635,62.4867253588613,38.));
#5984=CARTESIAN_POINT('Ctrl Pts',(41.4150926413892,62.9206514303181,38.));
#5985=CARTESIAN_POINT('Ctrl Pts',(41.6188649978616,63.1625011801094,38.));
#5986=CARTESIAN_POINT('Ctrl Pts',(42.0643495443749,63.5323654074303,38.));
#5987=CARTESIAN_POINT('Ctrl Pts',(42.398381143829,63.7105066153047,38.));
#5988=CARTESIAN_POINT('Ctrl Pts',(43.0349690410079,63.9313624698626,38.));
#5989=CARTESIAN_POINT('Ctrl Pts',(43.4594642227257,63.9999999999999,38.));
#5990=CARTESIAN_POINT('Ctrl Pts',(43.8178046004133,63.9999999999999,38.));
#5991=CARTESIAN_POINT('Origin',(-2.19535935928689E-13,63.9999999999997,
0.));
#5992=CARTESIAN_POINT('Origin',(88.,64.0000000000001,0.));
#5993=CARTESIAN_POINT('',(59.464274989274,64.,-38.));
#5994=CARTESIAN_POINT('Origin',(59.464274989274,64.,-8.));
#5995=CARTESIAN_POINT('',(43.8178046004133,63.9999999999999,-38.));
#5996=CARTESIAN_POINT('',(59.464274989274,64.,38.));
#5997=CARTESIAN_POINT('',(59.464274989274,64.,38.));
#5998=CARTESIAN_POINT('Origin',(59.464274989274,64.,8.));
#5999=CARTESIAN_POINT('',(-5.9999999999995,63.9999999999997,70.0000000000003));
#6000=CARTESIAN_POINT('Origin',(5.13675145228373E-13,63.9999999999998,70.0000000000002));
#6001=CARTESIAN_POINT('',(-70.0000000000004,63.9999999999995,-6.00000000000001));
#6002=CARTESIAN_POINT('Origin',(-70.0000000000004,63.9999999999995,0.));
#6003=CARTESIAN_POINT('',(5.99999999999955,63.9999999999998,-70.0000000000002));
#6004=CARTESIAN_POINT('Origin',(-4.63939629647707E-13,63.9999999999998,
-70.0000000000002));
#6005=CARTESIAN_POINT('Origin',(30.,-1.01376661467639E-14,0.));
#6006=CARTESIAN_POINT('',(-4.40872847693047E-15,-1.11022302462516E-13,36.));
#6007=CARTESIAN_POINT('Origin',(0.,-1.11022302462516E-13,0.));
#6008=CARTESIAN_POINT('',(30.,-8.11483249594263E-15,0.));
#6009=CARTESIAN_POINT('Origin',(0.,-1.11022302462516E-13,0.));
#6010=CARTESIAN_POINT('Origin',(0.,-1.11022302462516E-13,0.));
#6011=CARTESIAN_POINT('',(26.,-4.00000000000002,0.));
#6012=CARTESIAN_POINT('',(-25.9999999999999,-4.0000000000002,-3.18408167778311E-15));
#6013=CARTESIAN_POINT('Origin',(1.37209959955428E-14,-4.00000000000011,
0.));
#6014=CARTESIAN_POINT('Origin',(1.37209959955428E-14,-4.00000000000011,
0.));
#6015=CARTESIAN_POINT('',(30.,-8.11483249594263E-15,-3.67394039744206E-15));
#6016=CARTESIAN_POINT('Origin',(2.26992721413867E-12,-661.73832129271,0.));
#6017=CARTESIAN_POINT('',(-25.9999999999999,-30.0000000000003,-3.18408167778311E-15));
#6018=CARTESIAN_POINT('',(-25.9999999999977,-661.73832129271,-3.18408167778311E-15));
#6019=CARTESIAN_POINT('Origin',(1.02907469966573E-13,-30.0000000000001,
0.));
#6020=CARTESIAN_POINT('Origin',(26.,-30.,0.));
#6021=CARTESIAN_POINT('',(-23.9999999999997,-30.0000000000002,-2.93915231795363E-15));
#6022=CARTESIAN_POINT('Origin',(1.02907469966573E-13,-30.0000000000001,
0.));
#6023=CARTESIAN_POINT('Origin',(2.26992721413867E-12,-661.73832129271,0.));
#6024=CARTESIAN_POINT('',(-23.9999999999995,-80.0000000000003,-2.93915231795363E-15));
#6025=CARTESIAN_POINT('',(-23.9999999999975,-661.73832129271,-2.93915231795363E-15));
#6026=CARTESIAN_POINT('Origin',(2.74419919910861E-13,-80.0000000000001,
0.));
#6027=CARTESIAN_POINT('Origin',(24.,-80.0000000000001,0.));
#6028=CARTESIAN_POINT('',(-83.9999999999995,-80.0000000000005,-1.02870331128377E-14));
#6029=CARTESIAN_POINT('Origin',(2.74419919910862E-13,-80.0000000000003,
0.));
#6030=CARTESIAN_POINT('',(-71.9999999999997,-80.0000000000005,2.22475088246643E-13));
#6031=CARTESIAN_POINT('Origin',(-63.9999999999997,-80.0000000000004,2.23454805685961E-13));
#6032=CARTESIAN_POINT('',(-7.99999999999973,-80.0000000000002,64.));
#6033=CARTESIAN_POINT('Origin',(2.74419919910862E-13,-80.0000000000002,
64.));
#6034=CARTESIAN_POINT('',(56.0000000000003,-80.,-6.71344134497199E-13));
#6035=CARTESIAN_POINT('Origin',(64.0000000000003,-80.,-6.70364417057882E-13));
#6036=CARTESIAN_POINT('',(-7.99999999999973,-80.0000000000002,-64.));
#6037=CARTESIAN_POINT('Origin',(2.74419919910862E-13,-80.0000000000002,
-64.));
#6038=CARTESIAN_POINT('Origin',(2.26992721413867E-12,-661.73832129271,0.));
#6039=CARTESIAN_POINT('',(-83.9999999999995,-65.0000000000006,0.));
#6040=CARTESIAN_POINT('',(-83.9999999999975,-661.73832129271,-1.02870331128377E-14));
#6041=CARTESIAN_POINT('',(2.12679151814737E-13,-65.0000000000003,-83.9999999999998));
#6042=CARTESIAN_POINT('Origin',(2.22966184927575E-13,-65.0000000000003,
0.));
#6043=CARTESIAN_POINT('Origin',(2.22966184927575E-13,-65.0000000000003,
0.));
#6044=CARTESIAN_POINT('Origin',(84.,-63.9999999999999,0.));
#6045=CARTESIAN_POINT('',(2.09371367495766E-13,-64.0000000000002,-82.9999999999998));
#6046=CARTESIAN_POINT('Origin',(2.19535935928689E-13,-64.0000000000002,
0.));
#6047=CARTESIAN_POINT('',(-71.9999999999998,-64.0000000000005,2.23454805685961E-13));
#6048=CARTESIAN_POINT('Origin',(-63.9999999999998,-64.0000000000005,2.23454805685961E-13));
#6049=CARTESIAN_POINT('',(-7.99999999999978,-64.0000000000003,64.));
#6050=CARTESIAN_POINT('Origin',(2.1953593592869E-13,-64.0000000000002,64.));
#6051=CARTESIAN_POINT('',(56.0000000000002,-64.,-6.70364417057882E-13));
#6052=CARTESIAN_POINT('Origin',(64.0000000000002,-64.,-6.70364417057882E-13));
#6053=CARTESIAN_POINT('',(-7.99999999999978,-64.0000000000003,-64.));
#6054=CARTESIAN_POINT('Origin',(2.1953593592869E-13,-64.0000000000002,-64.));
#6055=CARTESIAN_POINT('',(-39.9999999999996,-64.0000000000002,-4.89858719658939E-15));
#6056=CARTESIAN_POINT('Origin',(2.19535935928689E-13,-64.0000000000001,
0.));
#6057=CARTESIAN_POINT('Origin',(2.26992721413867E-12,-661.73832129271,0.));
#6058=CARTESIAN_POINT('',(-39.9999999999998,-20.0000000000003,-4.89858719658939E-15));
#6059=CARTESIAN_POINT('',(-39.9999999999976,-661.73832129271,-4.89858719658939E-15));
#6060=CARTESIAN_POINT('',(6.44903518424829E-14,-20.0000000000001,39.9999999999999));
#6061=CARTESIAN_POINT('Origin',(6.86049799777153E-14,-20.0000000000001,
0.));
#6062=CARTESIAN_POINT('Origin',(6.86049799777153E-14,-20.0000000000001,
0.));
#6063=CARTESIAN_POINT('Origin',(6.93889390390723E-14,-20.0000000000001,
0.));
#6064=CARTESIAN_POINT('',(5.73849244848819E-14,-18.0000000000001,42.));
#6065=CARTESIAN_POINT('Origin',(6.42454224826534E-14,-20.0000000000001,
41.9999999999999));
#6066=CARTESIAN_POINT('Origin',(6.17444819799439E-14,-18.0000000000001,
0.));
#6067=CARTESIAN_POINT('Origin',(42.,-18.,0.));
#6068=CARTESIAN_POINT('',(5.6258156874715E-14,-18.0000000000001,47.9999999999999));
#6069=CARTESIAN_POINT('Origin',(6.17444819799439E-14,-18.0000000000001,
0.));
#6070=CARTESIAN_POINT('Origin',(3.46944695195361E-14,-10.0000000000001,
0.));
#6071=CARTESIAN_POINT('',(2.78364474443114E-14,-10.0000000000002,56.));
#6072=CARTESIAN_POINT('Origin',(2.88161648836289E-14,-10.0000000000001,
48.));
#6073=CARTESIAN_POINT('',(-56.0000000000001,-10.0000000000007,-6.85802207522519E-15));
#6074=CARTESIAN_POINT('Origin',(3.43024899888579E-14,-10.0000000000002,
0.));
#6075=CARTESIAN_POINT('Origin',(3.43024899888579E-14,-10.0000000000002,
0.));
#6076=CARTESIAN_POINT('Origin',(3.43024899888579E-14,-10.0000000000002,
0.));
#6077=CARTESIAN_POINT('Origin',(2.26992721413867E-12,-661.73832129271,0.));
#6078=CARTESIAN_POINT('',(-55.9999999999978,-661.73832129271,-6.85802207522519E-15));
#6079=CARTESIAN_POINT('Origin',(2.26992721413867E-12,-661.73832129271,0.));
#6080=CARTESIAN_POINT('',(89.1964124839111,65.9999999999999,-12.));
#6081=CARTESIAN_POINT('',(-90.0000000000005,79.9999999999994,-1.10218211923262E-14));
#6082=CARTESIAN_POINT('',(-89.999999999998,-661.73832129271,-1.10218211923262E-14));
#6083=CARTESIAN_POINT('Origin',(-2.74419919910861E-13,79.9999999999996,
0.));
#6084=CARTESIAN_POINT('',(89.1964124839111,65.9999999999999,12.));
#6085=CARTESIAN_POINT('Origin',(39.9999999999977,79.9999999999999,0.));
#6086=CARTESIAN_POINT('',(-2.79440971787365E-13,79.9999999999998,-40.999999999998));
#6087=CARTESIAN_POINT('Origin',(-2.74419919910861E-13,79.9999999999998,
0.));
#6088=CARTESIAN_POINT('',(-5.99999999999955,79.9999999999997,70.0000000000003));
#6089=CARTESIAN_POINT('Origin',(4.58791161246202E-13,79.9999999999997,70.0000000000003));
#6090=CARTESIAN_POINT('',(-70.0000000000005,79.9999999999995,-6.00000000000001));
#6091=CARTESIAN_POINT('Origin',(-70.0000000000006,79.9999999999994,0.));
#6092=CARTESIAN_POINT('',(5.99999999999949,79.9999999999997,-70.0000000000003));
#6093=CARTESIAN_POINT('Origin',(-5.1882361362988E-13,79.9999999999997,-70.0000000000003));
#6094=CARTESIAN_POINT('',(70.,79.9999999999999,6.00000000000001));
#6095=CARTESIAN_POINT('Origin',(70.,79.9999999999999,0.));
#6096=CARTESIAN_POINT('Origin',(2.26992721413867E-12,-661.73832129271,0.));
#6097=CARTESIAN_POINT('',(-39.9999999999983,78.9999999999997,0.));
#6098=CARTESIAN_POINT('',(-2.75888258108565E-13,78.9999999999998,-39.999999999998));
#6099=CARTESIAN_POINT('Origin',(-2.70989670911976E-13,78.9999999999998,
0.));
#6100=CARTESIAN_POINT('Origin',(-2.70989670911976E-13,78.9999999999998,
0.));
#6101=CARTESIAN_POINT('',(-39.9999999999982,71.9999999999997,-4.89858719658917E-15));
#6102=CARTESIAN_POINT('',(-39.9999999999957,-661.73832129271,-4.89858719658917E-15));
#6103=CARTESIAN_POINT('Origin',(-2.46977927919775E-13,71.9999999999998,
0.));
#6104=CARTESIAN_POINT('Origin',(44.,72.,0.));
#6105=CARTESIAN_POINT('',(-44.0000000000004,71.9999999999997,-5.38844591624837E-15));
#6106=CARTESIAN_POINT('Origin',(-2.46977927919775E-13,71.9999999999998,
0.));
#6107=CARTESIAN_POINT('Origin',(2.26992721413867E-12,-661.73832129271,0.));
#6108=CARTESIAN_POINT('',(-44.0000000000001,-2.50000000000014,-5.38844591624837E-15));
#6109=CARTESIAN_POINT('',(-43.9999999999978,-661.73832129271,-5.38844591624837E-15));
#6110=CARTESIAN_POINT('Origin',(8.57562249721397E-15,-2.50000000000006,
0.));
#6111=CARTESIAN_POINT('',(36.8781778291716,21.9999999999997,-24.));
#6112=CARTESIAN_POINT('',(36.8781778291716,21.9999999999997,24.));
#6113=CARTESIAN_POINT('Ctrl Pts',(36.8781778291716,21.9999999999997,-24.));
#6114=CARTESIAN_POINT('Ctrl Pts',(36.8781778291716,23.547692417105,-24.));
#6115=CARTESIAN_POINT('Ctrl Pts',(36.9785122566031,25.1334863360913,-23.8479816802424));
#6116=CARTESIAN_POINT('Ctrl Pts',(37.3739040154025,28.2623534606261,-23.2234342163971));
#6117=CARTESIAN_POINT('Ctrl Pts',(37.668184781229,29.8055820781137,-22.7511923092776));
#6118=CARTESIAN_POINT('Ctrl Pts',(38.3858791967795,32.7476022190956,-21.5182029027182));
#6119=CARTESIAN_POINT('Ctrl Pts',(38.8088904227423,34.1493429299749,-20.7564665668354));
#6120=CARTESIAN_POINT('Ctrl Pts',(39.6947646020434,36.7360406873461,-19.0075391135467));
#6121=CARTESIAN_POINT('Ctrl Pts',(40.1568366987602,37.9210704450902,-18.0200550518638));
#6122=CARTESIAN_POINT('Ctrl Pts',(41.0325054029201,40.0157721605676,-15.9253533363863));
#6123=CARTESIAN_POINT('Ctrl Pts',(41.4789748531813,41.0026054632418,-14.7424846218932));
#6124=CARTESIAN_POINT('Ctrl Pts',(42.3095898911624,42.7531938862499,-12.1550323282439));
#6125=CARTESIAN_POINT('Ctrl Pts',(42.6931404535345,43.5170818808236,-10.7503476715086));
#6126=CARTESIAN_POINT('Ctrl Pts',(43.3290028514715,44.7526497513758,-7.8020338794679));
#6127=CARTESIAN_POINT('Ctrl Pts',(43.5814918372967,45.2253213499122,-6.25551064938976));
#6128=CARTESIAN_POINT('Ctrl Pts',(43.9170909199956,45.8491089125422,-3.1252150936039));
#6129=CARTESIAN_POINT('Ctrl Pts',(44.,45.9999999999997,-1.54137641234701));
#6130=CARTESIAN_POINT('Ctrl Pts',(44.,45.9999999999997,1.54137641234701));
#6131=CARTESIAN_POINT('Ctrl Pts',(43.9170909199956,45.8491089125422,3.1252150936039));
#6132=CARTESIAN_POINT('Ctrl Pts',(43.5814918372967,45.2253213499122,6.25551064938976));
#6133=CARTESIAN_POINT('Ctrl Pts',(43.3290028514715,44.7526497513758,7.8020338794679));
#6134=CARTESIAN_POINT('Ctrl Pts',(42.6931404535345,43.5170818808236,10.7503476715086));
#6135=CARTESIAN_POINT('Ctrl Pts',(42.3095898911624,42.7531938862499,12.1550323282439));
#6136=CARTESIAN_POINT('Ctrl Pts',(41.4789748531813,41.0026054632418,14.7424846218932));
#6137=CARTESIAN_POINT('Ctrl Pts',(41.0325054029201,40.0157721605676,15.9253533363863));
#6138=CARTESIAN_POINT('Ctrl Pts',(40.1568366987602,37.9210704450902,18.0200550518638));
#6139=CARTESIAN_POINT('Ctrl Pts',(39.6947646020433,36.7360406873461,19.0075391135467));
#6140=CARTESIAN_POINT('Ctrl Pts',(38.8088904227423,34.1493429299749,20.7564665668354));
#6141=CARTESIAN_POINT('Ctrl Pts',(38.3858791967795,32.7476022190956,21.5182029027182));
#6142=CARTESIAN_POINT('Ctrl Pts',(37.668184781229,29.8055820781137,22.7511923092776));
#6143=CARTESIAN_POINT('Ctrl Pts',(37.3739040154025,28.2623534606261,23.2234342163971));
#6144=CARTESIAN_POINT('Ctrl Pts',(36.9785122566031,25.1334863360913,23.8479816802424));
#6145=CARTESIAN_POINT('Ctrl Pts',(36.8781778291716,23.547692417105,24.));
#6146=CARTESIAN_POINT('Ctrl Pts',(36.8781778291716,21.9999999999997,24.));
#6147=CARTESIAN_POINT('Ctrl Pts',(36.8781778291716,21.9999999999997,24.));
#6148=CARTESIAN_POINT('Ctrl Pts',(36.8781778291716,20.4523075828945,24.));
#6149=CARTESIAN_POINT('Ctrl Pts',(36.9785122566031,18.8665136639082,23.8479816802424));
#6150=CARTESIAN_POINT('Ctrl Pts',(37.3739040154025,15.7376465393734,23.2234342163972));
#6151=CARTESIAN_POINT('Ctrl Pts',(37.6681847812291,14.1944179218858,22.7511923092776));
#6152=CARTESIAN_POINT('Ctrl Pts',(38.3858791967795,11.2523977809039,21.5182029027182));
#6153=CARTESIAN_POINT('Ctrl Pts',(38.8088904227423,9.85065707002456,20.7564665668354));
#6154=CARTESIAN_POINT('Ctrl Pts',(39.6947646020434,7.26395931265332,19.0075391135467));
#6155=CARTESIAN_POINT('Ctrl Pts',(40.1568366987603,6.07892955490932,18.0200550518638));
#6156=CARTESIAN_POINT('Ctrl Pts',(41.0325054029202,3.98422783943184,15.9253533363864));
#6157=CARTESIAN_POINT('Ctrl Pts',(41.4789748531814,2.99739453675761,14.7424846218932));
#6158=CARTESIAN_POINT('Ctrl Pts',(42.3095898911626,1.24680611374955,12.1550323282439));
#6159=CARTESIAN_POINT('Ctrl Pts',(42.6931404535346,0.482918119175804,10.7503476715086));
#6160=CARTESIAN_POINT('Ctrl Pts',(43.3290028514716,-0.752649751376416,7.8020338794679));
#6161=CARTESIAN_POINT('Ctrl Pts',(43.5814918372968,-1.22532134991275,6.25551064938977));
#6162=CARTESIAN_POINT('Ctrl Pts',(43.9170909199958,-1.84910891254281,3.12521509360391));
#6163=CARTESIAN_POINT('Ctrl Pts',(44.0000000000001,-2.00000000000031,1.54137641234701));
#6164=CARTESIAN_POINT('Ctrl Pts',(44.0000000000001,-2.00000000000031,-1.54137641234702));
#6165=CARTESIAN_POINT('Ctrl Pts',(43.9170909199958,-1.84910891254281,-3.12521509360392));
#6166=CARTESIAN_POINT('Ctrl Pts',(43.5814918372968,-1.22532134991275,-6.25551064938977));
#6167=CARTESIAN_POINT('Ctrl Pts',(43.3290028514716,-0.752649751376415,-7.8020338794679));
#6168=CARTESIAN_POINT('Ctrl Pts',(42.6931404535346,0.482918119175804,-10.7503476715086));
#6169=CARTESIAN_POINT('Ctrl Pts',(42.3095898911626,1.24680611374955,-12.1550323282439));
#6170=CARTESIAN_POINT('Ctrl Pts',(41.4789748531814,2.99739453675761,-14.7424846218932));
#6171=CARTESIAN_POINT('Ctrl Pts',(41.0325054029202,3.98422783943184,-15.9253533363864));
#6172=CARTESIAN_POINT('Ctrl Pts',(40.1568366987603,6.07892955490932,-18.0200550518638));
#6173=CARTESIAN_POINT('Ctrl Pts',(39.6947646020434,7.26395931265332,-19.0075391135467));
#6174=CARTESIAN_POINT('Ctrl Pts',(38.8088904227423,9.85065707002456,-20.7564665668354));
#6175=CARTESIAN_POINT('Ctrl Pts',(38.3858791967795,11.2523977809039,-21.5182029027182));
#6176=CARTESIAN_POINT('Ctrl Pts',(37.6681847812291,14.1944179218858,-22.7511923092776));
#6177=CARTESIAN_POINT('Ctrl Pts',(37.3739040154025,15.7376465393734,-23.2234342163972));
#6178=CARTESIAN_POINT('Ctrl Pts',(36.9785122566031,18.8665136639082,-23.8479816802424));
#6179=CARTESIAN_POINT('Ctrl Pts',(36.8781778291716,20.4523075828945,-24.));
#6180=CARTESIAN_POINT('Ctrl Pts',(36.8781778291716,21.9999999999997,-24.));
#6181=CARTESIAN_POINT('Origin',(38.5,-2.50000000000001,0.));
#6182=CARTESIAN_POINT('',(3.86073232049693E-15,-2.50000000000006,38.5));
#6183=CARTESIAN_POINT('Origin',(8.57562249721397E-15,-2.50000000000006,
0.));
#6184=CARTESIAN_POINT('Origin',(0.,-1.11022302462516E-13,0.));
#6185=CARTESIAN_POINT('Origin',(-4.71489017671731E-15,-1.11022302462516E-13,
38.5));
#6186=CARTESIAN_POINT('Origin',(114.,21.9999999999997,0.));
#6187=CARTESIAN_POINT('',(130.,21.9999999999997,84.));
#6188=CARTESIAN_POINT('Origin',(130.,21.9999999999997,0.));
#6189=CARTESIAN_POINT('',(114.,21.9999999999997,84.));
#6190=CARTESIAN_POINT('',(114.,21.9999999999997,84.));
#6191=CARTESIAN_POINT('Origin',(114.,21.9999999999997,0.));
#6192=CARTESIAN_POINT('Origin',(114.,21.9999999999997,0.));
#6193=CARTESIAN_POINT('',(114.,21.9999999999995,-56.));
#6194=CARTESIAN_POINT('Origin',(114.,21.9999999999995,-64.));
#6195=CARTESIAN_POINT('',(114.,-42.0000000000003,8.));
#6196=CARTESIAN_POINT('Origin',(114.,-42.0000000000003,0.));
#6197=CARTESIAN_POINT('',(114.,22.0000000000004,72.));
#6198=CARTESIAN_POINT('Origin',(114.,22.0000000000004,64.));
#6199=CARTESIAN_POINT('',(114.,85.9999999999997,8.));
#6200=CARTESIAN_POINT('Origin',(114.,85.9999999999997,0.));
#6201=CARTESIAN_POINT('Origin',(130.,21.9999999999997,0.));
#6202=CARTESIAN_POINT('',(130.,21.9999999999995,-56.));
#6203=CARTESIAN_POINT('Origin',(130.,21.9999999999995,-64.));
#6204=CARTESIAN_POINT('',(130.,-42.0000000000003,8.));
#6205=CARTESIAN_POINT('Origin',(130.,-42.0000000000003,0.));
#6206=CARTESIAN_POINT('',(130.,22.0000000000004,72.));
#6207=CARTESIAN_POINT('Origin',(130.,22.0000000000004,64.));
#6208=CARTESIAN_POINT('',(130.,85.9999999999997,8.));
#6209=CARTESIAN_POINT('Origin',(130.,85.9999999999997,0.));
#6210=CARTESIAN_POINT('',(130.,21.9999999999997,24.));
#6211=CARTESIAN_POINT('Origin',(130.,21.9999999999997,0.));
#6212=CARTESIAN_POINT('Origin',(3.62800908907132E-5,21.9999999999997,-8.87342752119391E-6));
#6213=CARTESIAN_POINT('',(41.13395568512,21.9999999999999,38.));
#6214=CARTESIAN_POINT('',(41.1339720798708,21.9999999999999,-38.));
#6215=CARTESIAN_POINT('Origin',(41.1339720798708,21.9999999999999,-38.));
#6216=CARTESIAN_POINT('',(59.4642749892742,22.,-38.));
#6217=CARTESIAN_POINT('Origin',(81.5843122174847,22.,38.));
#6218=CARTESIAN_POINT('',(59.4642749892742,22.,38.));
#6219=CARTESIAN_POINT('Origin',(-90.0010000000005,21.9999999999997,0.));
#6220=CARTESIAN_POINT('',(-90.0010000000005,21.9999999999997,24.));
#6221=CARTESIAN_POINT('Origin',(91.3725830020305,85.9999999999997,0.));
#6222=CARTESIAN_POINT('',(91.3725830020305,85.9999999999997,8.));
#6223=CARTESIAN_POINT('Origin',(91.3725830020305,22.0000000000004,64.));
#6224=CARTESIAN_POINT('',(91.3725830020305,22.0000000000004,72.));
#6225=CARTESIAN_POINT('Origin',(91.3725830020305,-42.0000000000003,0.));
#6226=CARTESIAN_POINT('',(91.3725830020305,-42.0000000000003,8.));
#6227=CARTESIAN_POINT('Origin',(91.3725830020305,21.9999999999995,-64.));
#6228=CARTESIAN_POINT('',(91.3725830020305,21.9999999999995,-56.));
#6229=CARTESIAN_POINT('Origin',(1.41918261424034E-13,-41.3725830020307,
-64.));
#6230=CARTESIAN_POINT('',(-7.99999999999986,-41.3725830020308,-64.));
#6231=CARTESIAN_POINT('Origin',(64.0000000000001,-41.3725830020305,-6.70364417057882E-13));
#6232=CARTESIAN_POINT('',(56.0000000000001,-41.3725830020305,-6.71344134497199E-13));
#6233=CARTESIAN_POINT('Origin',(1.41918261424034E-13,-41.3725830020307,
64.));
#6234=CARTESIAN_POINT('',(-7.99999999999986,-41.3725830020307,64.));
#6235=CARTESIAN_POINT('Origin',(-63.9999999999999,-41.3725830020309,2.23454805685961E-13));
#6236=CARTESIAN_POINT('',(-71.9999999999999,-41.3725830020309,2.22475088246643E-13));
#6237=CARTESIAN_POINT('Origin',(70.,54.3948362858346,0.));
#6238=CARTESIAN_POINT('',(70.,57.9999999999999,6.00000000000001));
#6239=CARTESIAN_POINT('',(70.,54.3948362858346,6.00000000000001));
#6240=CARTESIAN_POINT('',(70.,57.9999999999999,-6.00000000000002));
#6241=CARTESIAN_POINT('Origin',(70.,57.9999999999999,0.));
#6242=CARTESIAN_POINT('Origin',(70.,57.9999999999999,0.));
#6243=CARTESIAN_POINT('Origin',(70.,655.255455313392,0.));
#6244=CARTESIAN_POINT('',(70.,54.3948362858346,0.));
#6245=CARTESIAN_POINT('',(69.9999999999999,655.255455313392,-1000.));
#6246=CARTESIAN_POINT('Origin',(-4.30991526433058E-13,54.3948362858343,
-70.0000000000002));
#6247=CARTESIAN_POINT('',(5.99999999999958,54.3948362858344,-70.0000000000002));
#6248=CARTESIAN_POINT('Origin',(-70.0000000000004,54.3948362858341,0.));
#6249=CARTESIAN_POINT('',(-70.0000000000004,54.3948362858341,-6.00000000000001));
#6250=CARTESIAN_POINT('Origin',(5.46623248443022E-13,54.3948362858343,70.0000000000002));
#6251=CARTESIAN_POINT('',(-5.99999999999947,54.3948362858343,70.0000000000002));
#6252=CARTESIAN_POINT('Origin',(59.4642749892765,-661.73832129271,-8.));
#6253=CARTESIAN_POINT('Origin',(59.4642749892765,-661.73832129271,8.));
#6254=CARTESIAN_POINT('Origin',(-2.70989670911976E-13,78.9999999999998,
0.));
#6255=CARTESIAN_POINT('Origin',(-2.7601072278848E-13,78.9999999999998,-40.999999999998));
#6256=CARTESIAN_POINT('Origin',(2.22966184927575E-13,-65.0000000000003,
0.));
#6257=CARTESIAN_POINT('Origin',(2.12801616494652E-13,-65.0000000000003,
-82.9999999999998));
#9644=UNCERTAINTY_MEASURE_WITH_UNIT(LENGTH_MEASURE(0.01),#9669,
'DISTANCE_ACCURACY_VALUE',
'Maximum model space distance between geometric entities at asserted c
onnectivities');
#9655=UNCERTAINTY_MEASURE_WITH_UNIT(LENGTH_MEASURE(0.01),#9669,
'DISTANCE_ACCURACY_VALUE',
'Maximum model space distance between geometric entities at asserted c
onnectivities');
#9657=(
GEOMETRIC_REPRESENTATION_CONTEXT(3)
GLOBAL_UNCERTAINTY_ASSIGNED_CONTEXT((#9644))
GLOBAL_UNIT_ASSIGNED_CONTEXT((#9669,#9671,#9672))
REPRESENTATION_CONTEXT('','3D')
);
#9668=(
GEOMETRIC_REPRESENTATION_CONTEXT(3)
GLOBAL_UNCERTAINTY_ASSIGNED_CONTEXT((#9655))
GLOBAL_UNIT_ASSIGNED_CONTEXT((#9669,#9671,#9672))
REPRESENTATION_CONTEXT('','3D')
);
#9669=(
LENGTH_UNIT()
NAMED_UNIT(*)
SI_UNIT(.MILLI.,.METRE.)
);
#9671=(
NAMED_UNIT(*)
PLANE_ANGLE_UNIT()
SI_UNIT($,.RADIAN.)
);
#9672=(
NAMED_UNIT(*)
SI_UNIT($,.STERADIAN.)
SOLID_ANGLE_UNIT()
);
#9674=SHAPE_DEFINITION_REPRESENTATION(#9686,#9712);
#9686=PRODUCT_DEFINITION_SHAPE('',$,#9725);
#9712=SHAPE_REPRESENTATION('',(#4015),#9657);
#9723=PRODUCT_DEFINITION_CONTEXT('part definition',#9761,'design');
#9725=PRODUCT_DEFINITION('2026-10-04-08-13-48-880','VALVE_BODY',#9737,#9723);
#9737=PRODUCT_DEFINITION_FORMATION('',$,#9764);
#9761=APPLICATION_CONTEXT(
'Core Data for Automotive Mechanical Design Process');
#9762=PRODUCT_CONTEXT('part definition',#9761,'mechanical');
#9764=PRODUCT('2026-10-04-08-13-48-880','VALVE_BODY','PART',(#9762));
#9775=PRESENTATION_STYLE_ASSIGNMENT((#9776));
#9776=SURFACE_STYLE_USAGE(.BOTH.,#9777);
#9777=SURFACE_SIDE_STYLE('',(#9778));
#9778=SURFACE_STYLE_FILL_AREA(#9779);
#9779=FILL_AREA_STYLE('Steel - Satin',(#9780));
#9780=FILL_AREA_STYLE_COLOUR('Steel - Satin',#9781);
#9781=COLOUR_RGB('Steel - Satin', 0.09019608, 0.27058824, 0.51372549);
ENDSEC;
END-ISO-10303-21;
